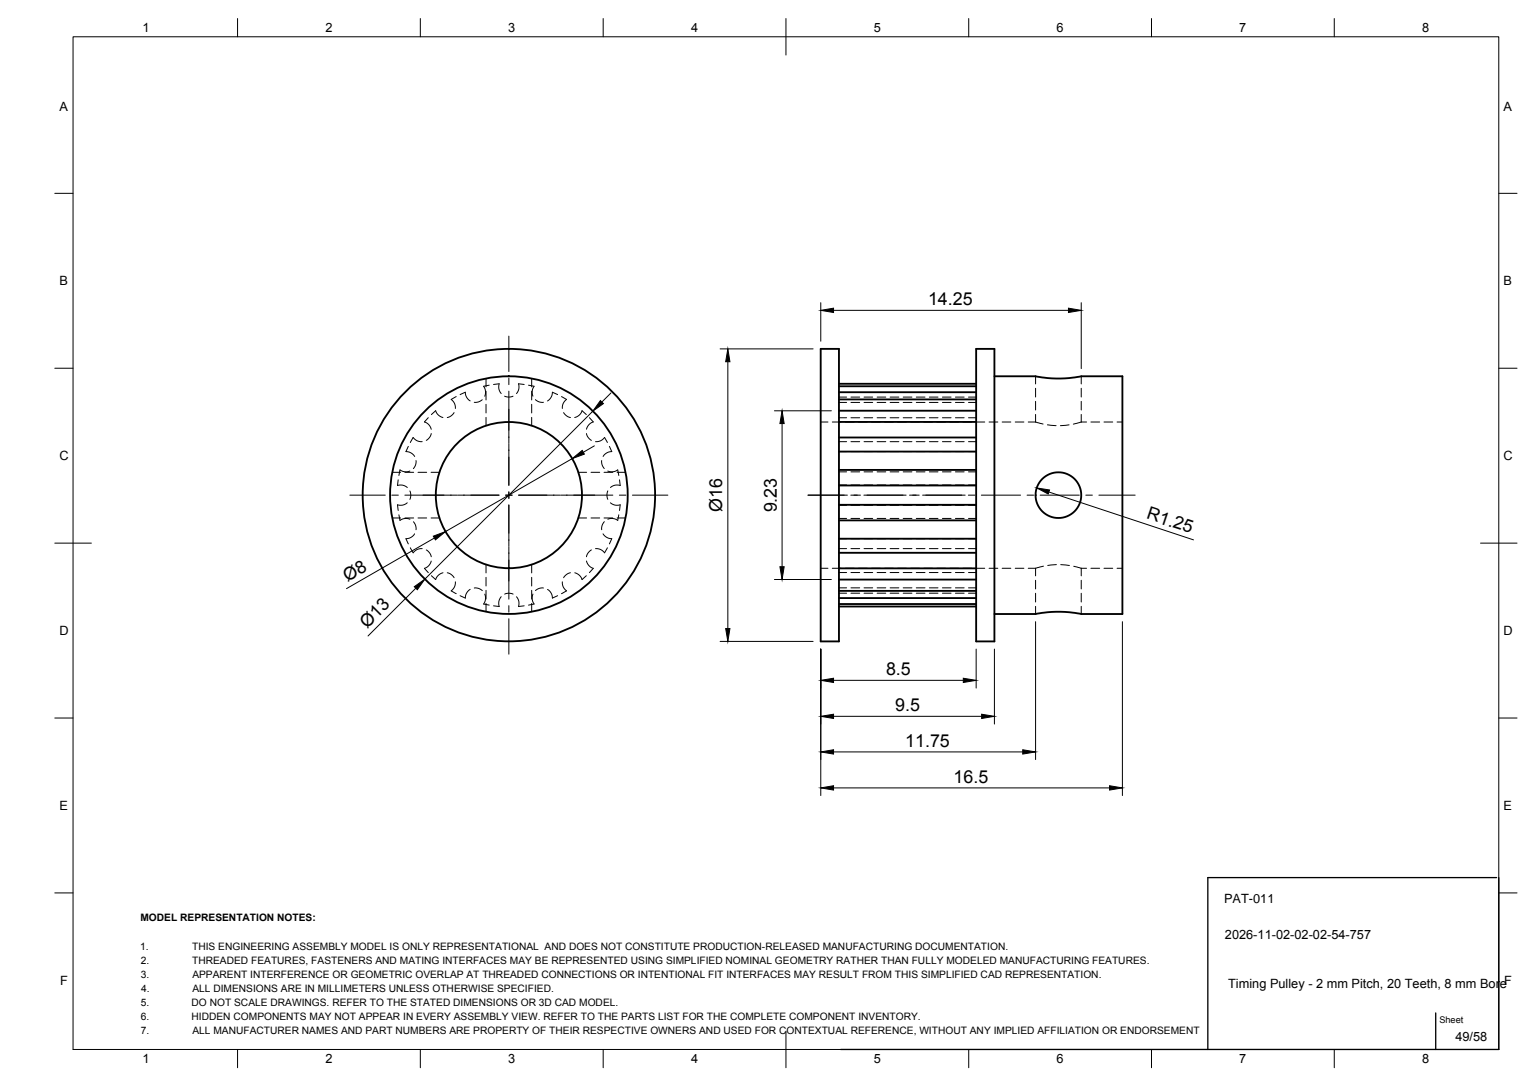
ISO-10303-21;
HEADER;
/* Generated by software containing ST-Developer
 * from STEP Tools, Inc. (www.steptools.com) 
 */

FILE_DESCRIPTION(
/* description */ ('Belt tension measurement rig'),
/* implementation_level */ '2;1');

FILE_NAME(
/* name */ 'Timing Pulley - 2 mm Pitch, 20 Teeth, 8 mm Bore.step',
/* time_stamp */ '2026-10-28T03:24:44-07:00',
/* author */ (''),
/* organization */ (''),
/* preprocessor_version */ 'ST-DEVELOPER v20.2',
/* originating_system */ 'Autodesk Translation Framework v15.17.0.0',
/* authorisation */ '');

FILE_SCHEMA (('AUTOMOTIVE_DESIGN { 1 0 10303 214 3 1 1 }'));
ENDSEC;

DATA;
#10=MECHANICAL_DESIGN_GEOMETRIC_PRESENTATION_REPRESENTATION('',(#750),#23587);
#531=B_SPLINE_CURVE_WITH_KNOTS('',3,(#21553,#21554,#21555,#21556,#21557,
#21558,#21559,#21560,#21561,#21562),.UNSPECIFIED.,.F.,.F.,(4,2,2,2,4),(0.566550474129931,
0.613761886174531,0.66097329821913,0.708186965196186,0.755400632173242),
 .UNSPECIFIED.);
#532=B_SPLINE_CURVE_WITH_KNOTS('',3,(#21564,#21565,#21566,#21567,#21568,
#21569,#21570,#21571,#21572,#21573,#21574,#21575,#21576,#21577,#21578,#21579,
#21580,#21581),.UNSPECIFIED.,.F.,.F.,(4,2,2,2,2,2,2,2,4),(0.18885015804331,
0.23606157008791,0.283272982132509,0.330486649109565,0.377700316086621,
0.424913983063677,0.472127650040732,0.519339062085332,0.566550474129931),
 .UNSPECIFIED.);
#533=B_SPLINE_CURVE_WITH_KNOTS('',3,(#21582,#21583,#21584,#21585,#21586,
#21587,#21588,#21589,#21590,#21591),.UNSPECIFIED.,.F.,.F.,(4,2,2,2,4),(0.755400632173242,
0.802614299150298,0.849827966127353,0.897039378171953,0.944250790216552),
 .UNSPECIFIED.);
#534=B_SPLINE_CURVE_WITH_KNOTS('',3,(#21595,#21596,#21597,#21598,#21599,
#21600,#21601,#21602,#21603,#21604),.UNSPECIFIED.,.F.,.F.,(4,2,2,2,4),(0.189723673274825,
0.237146208024627,0.28456874277443,0.33200804466204,0.37944734654965),
 .UNSPECIFIED.);
#535=B_SPLINE_CURVE_WITH_KNOTS('',3,(#21606,#21607,#21608,#21609,#21610,
#21611,#21612,#21613,#21614,#21615),.UNSPECIFIED.,.F.,.F.,(4,2,2,2,4),(0.,
0.0474393018876097,0.0948786037752193,0.142301138525022,0.189723673274825),
 .UNSPECIFIED.);
#536=B_SPLINE_CURVE_WITH_KNOTS('',3,(#21617,#21618,#21619,#21620,#21621,
#21622,#21623,#21624,#21625,#21626),.UNSPECIFIED.,.F.,.F.,(4,2,2,2,4),(0.569171019824474,
0.616593554574277,0.66401608932408,0.711455391211689,0.758894693099299),
 .UNSPECIFIED.);
#537=B_SPLINE_CURVE_WITH_KNOTS('',3,(#21627,#21628,#21629,#21630,#21631,
#21632,#21633,#21634,#21635,#21636),.UNSPECIFIED.,.F.,.F.,(4,2,2,2,4),(0.37944734654965,
0.426886648437259,0.474325950324869,0.521748485074671,0.569171019824474),
 .UNSPECIFIED.);
#538=B_SPLINE_CURVE_WITH_KNOTS('',3,(#21640,#21641,#21642,#21643,#21644,
#21645,#21646,#21647,#21648,#21649,#21650,#21651,#21652,#21653,#21654,#21655,
#21656,#21657),.UNSPECIFIED.,.F.,.F.,(4,2,2,2,2,2,2,2,4),(0.,0.0474393018876097,
0.0948786037752194,0.142301138525022,0.189723673274825,0.237146208024628,
0.28456874277443,0.33200804466204,0.37944734654965),.UNSPECIFIED.);
#539=B_SPLINE_CURVE_WITH_KNOTS('',3,(#21658,#21659,#21660,#21661,#21662,
#21663,#21664,#21665,#21666,#21667,#21668,#21669,#21670,#21671,#21672,#21673,
#21674,#21675),.UNSPECIFIED.,.F.,.F.,(4,2,2,2,2,2,2,2,4),(0.37944734654965,
0.426886648437259,0.474325950324869,0.521748485074672,0.569171019824474,
0.616593554574277,0.66401608932408,0.711455391211689,0.758894693099299),
 .UNSPECIFIED.);
#540=B_SPLINE_CURVE_WITH_KNOTS('',3,(#21679,#21680,#21681,#21682,#21683,
#21684,#21685,#21686,#21687,#21688),.UNSPECIFIED.,.F.,.F.,(4,2,2,2,4),(0.566550474129931,
0.613761886174531,0.66097329821913,0.708186965196186,0.755400632173242),
 .UNSPECIFIED.);
#541=B_SPLINE_CURVE_WITH_KNOTS('',3,(#21690,#21691,#21692,#21693,#21694,
#21695,#21696,#21697,#21698,#21699,#21700,#21701,#21702,#21703,#21704,#21705,
#21706,#21707),.UNSPECIFIED.,.F.,.F.,(4,2,2,2,2,2,2,2,4),(0.188850158043311,
0.23606157008791,0.283272982132509,0.330486649109565,0.377700316086621,
0.424913983063677,0.472127650040733,0.519339062085332,0.566550474129931),
 .UNSPECIFIED.);
#542=B_SPLINE_CURVE_WITH_KNOTS('',3,(#21708,#21709,#21710,#21711,#21712,
#21713,#21714,#21715,#21716,#21717),.UNSPECIFIED.,.F.,.F.,(4,2,2,2,4),(0.755400632173242,
0.802614299150298,0.849827966127354,0.897039378171953,0.944250790216552),
 .UNSPECIFIED.);
#543=B_SPLINE_CURVE_WITH_KNOTS('',3,(#21727,#21728,#21729,#21730,#21731,
#21732,#21733,#21734,#21735,#21736,#21737,#21738,#21739,#21740,#21741,#21742,
#21743,#21744),.UNSPECIFIED.,.F.,.F.,(4,2,2,2,2,2,2,2,4),(0.18885015804331,
0.23606157008791,0.283272982132509,0.330486649109565,0.377700316086621,
0.424913983063677,0.472127650040732,0.519339062085332,0.566550474129931),
 .UNSPECIFIED.);
#544=B_SPLINE_CURVE_WITH_KNOTS('',3,(#21746,#21747,#21748,#21749,#21750,
#21751,#21752,#21753,#21754,#21755),.UNSPECIFIED.,.F.,.F.,(4,2,2,2,4),(0.566550474129931,
0.613761886174531,0.66097329821913,0.708186965196186,0.755400632173242),
 .UNSPECIFIED.);
#545=B_SPLINE_CURVE_WITH_KNOTS('',3,(#21756,#21757,#21758,#21759,#21760,
#21761,#21762,#21763,#21764,#21765),.UNSPECIFIED.,.F.,.F.,(4,2,2,2,4),(0.755400632173242,
0.802614299150298,0.849827966127353,0.897039378171953,0.944250790216552),
 .UNSPECIFIED.);
#546=B_SPLINE_CURVE_WITH_KNOTS('',3,(#21768,#21769,#21770,#21771,#21772,
#21773,#21774,#21775,#21776,#21777,#21778,#21779,#21780,#21781,#21782,#21783,
#21784,#21785),.UNSPECIFIED.,.F.,.F.,(4,2,2,2,2,2,2,2,4),(0.188850158043311,
0.23606157008791,0.283272982132509,0.330486649109565,0.377700316086621,
0.424913983063677,0.472127650040733,0.519339062085332,0.566550474129932),
 .UNSPECIFIED.);
#547=B_SPLINE_CURVE_WITH_KNOTS('',3,(#21787,#21788,#21789,#21790,#21791,
#21792,#21793,#21794,#21795,#21796),.UNSPECIFIED.,.F.,.F.,(4,2,2,2,4),(0.566550474129932,
0.613761886174531,0.66097329821913,0.708186965196186,0.755400632173242),
 .UNSPECIFIED.);
#548=B_SPLINE_CURVE_WITH_KNOTS('',3,(#21797,#21798,#21799,#21800,#21801,
#21802,#21803,#21804,#21805,#21806),.UNSPECIFIED.,.F.,.F.,(4,2,2,2,4),(0.755400632173242,
0.802614299150298,0.849827966127354,0.897039378171953,0.944250790216552),
 .UNSPECIFIED.);
#549=B_SPLINE_CURVE_WITH_KNOTS('',3,(#21811,#21812,#21813,#21814,#21815,
#21816,#21817,#21818,#21819,#21820,#21821,#21822,#21823,#21824,#21825,#21826,
#21827,#21828),.UNSPECIFIED.,.F.,.F.,(4,2,2,2,2,2,2,2,4),(0.,0.0474393018876097,
0.0948786037752193,0.142301138525022,0.189723673274825,0.237146208024627,
0.28456874277443,0.33200804466204,0.37944734654965),.UNSPECIFIED.);
#550=B_SPLINE_CURVE_WITH_KNOTS('',3,(#21829,#21830,#21831,#21832,#21833,
#21834,#21835,#21836,#21837,#21838,#21839,#21840,#21841,#21842,#21843,#21844,
#21845,#21846),.UNSPECIFIED.,.F.,.F.,(4,2,2,2,2,2,2,2,4),(0.37944734654965,
0.426886648437259,0.474325950324869,0.521748485074672,0.569171019824474,
0.616593554574277,0.66401608932408,0.711455391211689,0.758894693099299),
 .UNSPECIFIED.);
#551=B_SPLINE_CURVE_WITH_KNOTS('',3,(#21850,#21851,#21852,#21853,#21854,
#21855,#21856,#21857,#21858,#21859,#21860,#21861,#21862,#21863,#21864,#21865,
#21866,#21867),.UNSPECIFIED.,.F.,.F.,(4,2,2,2,2,2,2,2,4),(0.,0.0474393018876097,
0.0948786037752194,0.142301138525022,0.189723673274825,0.237146208024627,
0.28456874277443,0.33200804466204,0.37944734654965),.UNSPECIFIED.);
#552=B_SPLINE_CURVE_WITH_KNOTS('',3,(#21868,#21869,#21870,#21871,#21872,
#21873,#21874,#21875,#21876,#21877,#21878,#21879,#21880,#21881,#21882,#21883,
#21884,#21885),.UNSPECIFIED.,.F.,.F.,(4,2,2,2,2,2,2,2,4),(0.37944734654965,
0.426886648437259,0.474325950324869,0.521748485074672,0.569171019824474,
0.616593554574277,0.66401608932408,0.711455391211689,0.758894693099299),
 .UNSPECIFIED.);
#625=SHAPE_REPRESENTATION_RELATIONSHIP('SRR','None',#23875,#680);
#680=ADVANCED_BREP_SHAPE_REPRESENTATION('',(#818),#23573);
#750=STYLED_ITEM('',(#24225),#818);
#818=MANIFOLD_SOLID_BREP('Body1',#12257);
#995=FACE_BOUND('',#2703,.T.);
#996=FACE_BOUND('',#2704,.T.);
#997=FACE_BOUND('',#2705,.T.);
#998=FACE_BOUND('',#2709,.T.);
#999=FACE_BOUND('',#2710,.T.);
#1000=FACE_BOUND('',#2711,.T.);
#1001=FACE_BOUND('',#2713,.T.);
#1002=FACE_BOUND('',#2715,.T.);
#1003=FACE_BOUND('',#2718,.T.);
#1004=FACE_BOUND('',#2720,.T.);
#1005=FACE_BOUND('',#2723,.T.);
#1294=PLANE('',#13882);
#1295=PLANE('',#13883);
#1296=PLANE('',#13927);
#1297=PLANE('',#13928);
#1298=PLANE('',#13972);
#1830=FACE_OUTER_BOUND('',#2700,.T.);
#1831=FACE_OUTER_BOUND('',#2701,.T.);
#1832=FACE_OUTER_BOUND('',#2702,.T.);
#1833=FACE_OUTER_BOUND('',#2706,.T.);
#1834=FACE_OUTER_BOUND('',#2707,.T.);
#1835=FACE_OUTER_BOUND('',#2708,.T.);
#1836=FACE_OUTER_BOUND('',#2712,.T.);
#1837=FACE_OUTER_BOUND('',#2714,.T.);
#1838=FACE_OUTER_BOUND('',#2716,.T.);
#1839=FACE_OUTER_BOUND('',#2717,.T.);
#1840=FACE_OUTER_BOUND('',#2719,.T.);
#1841=FACE_OUTER_BOUND('',#2721,.T.);
#1842=FACE_OUTER_BOUND('',#2722,.T.);
#1843=FACE_OUTER_BOUND('',#2724,.T.);
#1844=FACE_OUTER_BOUND('',#2725,.T.);
#1845=FACE_OUTER_BOUND('',#2726,.T.);
#1846=FACE_OUTER_BOUND('',#2727,.T.);
#1847=FACE_OUTER_BOUND('',#2728,.T.);
#1848=FACE_OUTER_BOUND('',#2729,.T.);
#1849=FACE_OUTER_BOUND('',#2730,.T.);
#1850=FACE_OUTER_BOUND('',#2731,.T.);
#1851=FACE_OUTER_BOUND('',#2732,.T.);
#1852=FACE_OUTER_BOUND('',#2733,.T.);
#1853=FACE_OUTER_BOUND('',#2734,.T.);
#1854=FACE_OUTER_BOUND('',#2735,.T.);
#1855=FACE_OUTER_BOUND('',#2736,.T.);
#1856=FACE_OUTER_BOUND('',#2737,.T.);
#1857=FACE_OUTER_BOUND('',#2738,.T.);
#1858=FACE_OUTER_BOUND('',#2739,.T.);
#1859=FACE_OUTER_BOUND('',#2740,.T.);
#1860=FACE_OUTER_BOUND('',#2741,.T.);
#1861=FACE_OUTER_BOUND('',#2742,.T.);
#1862=FACE_OUTER_BOUND('',#2743,.T.);
#1863=FACE_OUTER_BOUND('',#2744,.T.);
#1864=FACE_OUTER_BOUND('',#2745,.T.);
#1865=FACE_OUTER_BOUND('',#2746,.T.);
#1866=FACE_OUTER_BOUND('',#2747,.T.);
#1867=FACE_OUTER_BOUND('',#2748,.T.);
#1868=FACE_OUTER_BOUND('',#2749,.T.);
#1869=FACE_OUTER_BOUND('',#2750,.T.);
#1870=FACE_OUTER_BOUND('',#2751,.T.);
#1871=FACE_OUTER_BOUND('',#2752,.T.);
#1872=FACE_OUTER_BOUND('',#2753,.T.);
#1873=FACE_OUTER_BOUND('',#2754,.T.);
#1874=FACE_OUTER_BOUND('',#2755,.T.);
#1875=FACE_OUTER_BOUND('',#2756,.T.);
#1876=FACE_OUTER_BOUND('',#2757,.T.);
#1877=FACE_OUTER_BOUND('',#2758,.T.);
#1878=FACE_OUTER_BOUND('',#2759,.T.);
#1879=FACE_OUTER_BOUND('',#2760,.T.);
#1880=FACE_OUTER_BOUND('',#2761,.T.);
#1881=FACE_OUTER_BOUND('',#2762,.T.);
#1882=FACE_OUTER_BOUND('',#2763,.T.);
#2700=EDGE_LOOP('',(#10004,#10005,#10006,#10007,#10008,#10009,#10010,#10011,
#10012));
#2701=EDGE_LOOP('',(#10013,#10014,#10015,#10016,#10017,#10018,#10019));
#2702=EDGE_LOOP('',(#10020,#10021,#10022,#10023,#10024,#10025,#10026,#10027,
#10028));
#2703=EDGE_LOOP('',(#10029,#10030,#10031));
#2704=EDGE_LOOP('',(#10032,#10033,#10034));
#2705=EDGE_LOOP('',(#10035,#10036,#10037));
#2706=EDGE_LOOP('',(#10038,#10039,#10040,#10041,#10042,#10043,#10044));
#2707=EDGE_LOOP('',(#10045,#10046,#10047,#10048,#10049,#10050,#10051));
#2708=EDGE_LOOP('',(#10052,#10053,#10054,#10055,#10056,#10057,#10058,#10059,
#10060,#10061));
#2709=EDGE_LOOP('',(#10062,#10063));
#2710=EDGE_LOOP('',(#10064,#10065));
#2711=EDGE_LOOP('',(#10066,#10067));
#2712=EDGE_LOOP('',(#10068));
#2713=EDGE_LOOP('',(#10069));
#2714=EDGE_LOOP('',(#10070));
#2715=EDGE_LOOP('',(#10071,#10072,#10073,#10074,#10075,#10076,#10077,#10078,
#10079,#10080,#10081,#10082,#10083,#10084,#10085,#10086,#10087,#10088,#10089,
#10090,#10091,#10092,#10093,#10094,#10095,#10096,#10097,#10098,#10099,#10100,
#10101,#10102,#10103,#10104,#10105,#10106,#10107,#10108,#10109,#10110));
#2716=EDGE_LOOP('',(#10111,#10112,#10113,#10114));
#2717=EDGE_LOOP('',(#10115));
#2718=EDGE_LOOP('',(#10116));
#2719=EDGE_LOOP('',(#10117));
#2720=EDGE_LOOP('',(#10118,#10119,#10120,#10121,#10122,#10123,#10124,#10125,
#10126,#10127,#10128,#10129,#10130,#10131,#10132,#10133,#10134,#10135,#10136,
#10137,#10138,#10139,#10140,#10141,#10142,#10143,#10144,#10145,#10146,#10147,
#10148,#10149,#10150,#10151,#10152,#10153,#10154,#10155,#10156,#10157));
#2721=EDGE_LOOP('',(#10158,#10159,#10160,#10161));
#2722=EDGE_LOOP('',(#10162));
#2723=EDGE_LOOP('',(#10163));
#2724=EDGE_LOOP('',(#10164,#10165,#10166,#10167));
#2725=EDGE_LOOP('',(#10168,#10169,#10170,#10171));
#2726=EDGE_LOOP('',(#10172,#10173,#10174,#10175));
#2727=EDGE_LOOP('',(#10176,#10177,#10178,#10179));
#2728=EDGE_LOOP('',(#10180,#10181,#10182,#10183));
#2729=EDGE_LOOP('',(#10184,#10185,#10186,#10187));
#2730=EDGE_LOOP('',(#10188,#10189,#10190,#10191));
#2731=EDGE_LOOP('',(#10192,#10193,#10194,#10195));
#2732=EDGE_LOOP('',(#10196,#10197,#10198,#10199));
#2733=EDGE_LOOP('',(#10200,#10201,#10202,#10203));
#2734=EDGE_LOOP('',(#10204,#10205,#10206,#10207));
#2735=EDGE_LOOP('',(#10208,#10209,#10210,#10211));
#2736=EDGE_LOOP('',(#10212,#10213,#10214,#10215));
#2737=EDGE_LOOP('',(#10216,#10217,#10218,#10219));
#2738=EDGE_LOOP('',(#10220,#10221,#10222,#10223));
#2739=EDGE_LOOP('',(#10224,#10225,#10226,#10227));
#2740=EDGE_LOOP('',(#10228,#10229,#10230,#10231));
#2741=EDGE_LOOP('',(#10232,#10233,#10234,#10235));
#2742=EDGE_LOOP('',(#10236,#10237,#10238,#10239));
#2743=EDGE_LOOP('',(#10240,#10241,#10242,#10243));
#2744=EDGE_LOOP('',(#10244,#10245,#10246,#10247));
#2745=EDGE_LOOP('',(#10248,#10249,#10250,#10251));
#2746=EDGE_LOOP('',(#10252,#10253,#10254,#10255));
#2747=EDGE_LOOP('',(#10256,#10257,#10258,#10259));
#2748=EDGE_LOOP('',(#10260,#10261,#10262,#10263));
#2749=EDGE_LOOP('',(#10264,#10265,#10266,#10267));
#2750=EDGE_LOOP('',(#10268,#10269,#10270,#10271));
#2751=EDGE_LOOP('',(#10272,#10273,#10274,#10275));
#2752=EDGE_LOOP('',(#10276,#10277,#10278,#10279));
#2753=EDGE_LOOP('',(#10280,#10281,#10282,#10283));
#2754=EDGE_LOOP('',(#10284,#10285,#10286,#10287));
#2755=EDGE_LOOP('',(#10288,#10289,#10290,#10291));
#2756=EDGE_LOOP('',(#10292,#10293,#10294,#10295));
#2757=EDGE_LOOP('',(#10296,#10297,#10298,#10299));
#2758=EDGE_LOOP('',(#10300,#10301,#10302,#10303));
#2759=EDGE_LOOP('',(#10304,#10305,#10306,#10307));
#2760=EDGE_LOOP('',(#10308,#10309,#10310,#10311));
#2761=EDGE_LOOP('',(#10312,#10313,#10314,#10315));
#2762=EDGE_LOOP('',(#10316,#10317,#10318,#10319));
#2763=EDGE_LOOP('',(#10320,#10321,#10322,#10323));
#3507=LINE('',#21593,#4258);
#3508=LINE('',#21677,#4259);
#3509=LINE('',#21721,#4260);
#3510=LINE('',#21723,#4261);
#3511=LINE('',#21809,#4262);
#3512=LINE('',#21886,#4263);
#3513=LINE('',#21890,#4264);
#3514=LINE('',#21892,#4265);
#3515=LINE('',#21981,#4266);
#3516=LINE('',#22069,#4267);
#3517=LINE('',#22072,#4268);
#3518=LINE('',#22073,#4269);
#3519=LINE('',#22075,#4270);
#3520=LINE('',#22077,#4271);
#3521=LINE('',#22079,#4272);
#3522=LINE('',#22081,#4273);
#3523=LINE('',#22083,#4274);
#3524=LINE('',#22085,#4275);
#3525=LINE('',#22087,#4276);
#3526=LINE('',#22089,#4277);
#3527=LINE('',#22091,#4278);
#3528=LINE('',#22093,#4279);
#3529=LINE('',#22095,#4280);
#3530=LINE('',#22097,#4281);
#3531=LINE('',#22099,#4282);
#3532=LINE('',#22101,#4283);
#3533=LINE('',#22103,#4284);
#3534=LINE('',#22105,#4285);
#3535=LINE('',#22107,#4286);
#3536=LINE('',#22109,#4287);
#3537=LINE('',#22111,#4288);
#3538=LINE('',#22113,#4289);
#3539=LINE('',#22115,#4290);
#3540=LINE('',#22117,#4291);
#3541=LINE('',#22119,#4292);
#3542=LINE('',#22121,#4293);
#3543=LINE('',#22123,#4294);
#3544=LINE('',#22125,#4295);
#3545=LINE('',#22127,#4296);
#3546=LINE('',#22129,#4297);
#3547=LINE('',#22131,#4298);
#3548=LINE('',#22133,#4299);
#3549=LINE('',#22135,#4300);
#3550=LINE('',#22137,#4301);
#3551=LINE('',#22139,#4302);
#3552=LINE('',#22141,#4303);
#3553=LINE('',#22143,#4304);
#3554=LINE('',#22145,#4305);
#3555=LINE('',#22147,#4306);
#3556=LINE('',#22149,#4307);
#4258=VECTOR('',#17050,0.125);
#4259=VECTOR('',#17053,0.125);
#4260=VECTOR('',#17058,0.65);
#4261=VECTOR('',#17059,0.65);
#4262=VECTOR('',#17064,0.125);
#4263=VECTOR('',#17067,0.125);
#4264=VECTOR('',#17072,0.4);
#4265=VECTOR('',#17073,0.4);
#4266=VECTOR('',#17166,0.8);
#4267=VECTOR('',#17257,0.8);
#4268=VECTOR('',#17262,1.);
#4269=VECTOR('',#17263,1.);
#4270=VECTOR('',#17266,1.);
#4271=VECTOR('',#17269,1.);
#4272=VECTOR('',#17272,1.);
#4273=VECTOR('',#17275,1.);
#4274=VECTOR('',#17278,1.);
#4275=VECTOR('',#17281,1.);
#4276=VECTOR('',#17284,1.);
#4277=VECTOR('',#17287,1.);
#4278=VECTOR('',#17290,1.);
#4279=VECTOR('',#17293,1.);
#4280=VECTOR('',#17296,1.);
#4281=VECTOR('',#17299,1.);
#4282=VECTOR('',#17302,1.);
#4283=VECTOR('',#17305,1.);
#4284=VECTOR('',#17308,1.);
#4285=VECTOR('',#17311,1.);
#4286=VECTOR('',#17314,1.);
#4287=VECTOR('',#17317,1.);
#4288=VECTOR('',#17320,1.);
#4289=VECTOR('',#17323,1.);
#4290=VECTOR('',#17326,1.);
#4291=VECTOR('',#17329,1.);
#4292=VECTOR('',#17332,1.);
#4293=VECTOR('',#17335,1.);
#4294=VECTOR('',#17338,1.);
#4295=VECTOR('',#17341,1.);
#4296=VECTOR('',#17344,1.);
#4297=VECTOR('',#17347,1.);
#4298=VECTOR('',#17350,1.);
#4299=VECTOR('',#17353,1.);
#4300=VECTOR('',#17356,1.);
#4301=VECTOR('',#17359,1.);
#4302=VECTOR('',#17362,1.);
#4303=VECTOR('',#17365,1.);
#4304=VECTOR('',#17368,1.);
#4305=VECTOR('',#17371,1.);
#4306=VECTOR('',#17374,1.);
#4307=VECTOR('',#17377,1.);
#4924=CIRCLE('',#13875,0.65);
#4925=CIRCLE('',#13876,0.65);
#4926=CIRCLE('',#13880,0.4);
#4927=CIRCLE('',#13881,0.4);
#4928=CIRCLE('',#13884,0.8);
#4929=CIRCLE('',#13885,0.0555);
#4930=CIRCLE('',#13886,0.611219772367581);
#4931=CIRCLE('',#13887,0.0555);
#4932=CIRCLE('',#13888,0.611219772367581);
#4933=CIRCLE('',#13889,0.0555);
#4934=CIRCLE('',#13890,0.611219772367581);
#4935=CIRCLE('',#13891,0.0555);
#4936=CIRCLE('',#13892,0.611219772367581);
#4937=CIRCLE('',#13893,0.0555);
#4938=CIRCLE('',#13894,0.611219772367581);
#4939=CIRCLE('',#13895,0.0555);
#4940=CIRCLE('',#13896,0.611219772367581);
#4941=CIRCLE('',#13897,0.0555);
#4942=CIRCLE('',#13898,0.611219772367581);
#4943=CIRCLE('',#13899,0.0555);
#4944=CIRCLE('',#13900,0.611219772367581);
#4945=CIRCLE('',#13901,0.0555);
#4946=CIRCLE('',#13902,0.611219772367581);
#4947=CIRCLE('',#13903,0.0555);
#4948=CIRCLE('',#13904,0.611219772367581);
#4949=CIRCLE('',#13905,0.0555);
#4950=CIRCLE('',#13906,0.611219772367581);
#4951=CIRCLE('',#13907,0.0555);
#4952=CIRCLE('',#13908,0.611219772367581);
#4953=CIRCLE('',#13909,0.0555);
#4954=CIRCLE('',#13910,0.611219772367581);
#4955=CIRCLE('',#13911,0.0555);
#4956=CIRCLE('',#13912,0.611219772367581);
#4957=CIRCLE('',#13913,0.0555);
#4958=CIRCLE('',#13914,0.611219772367581);
#4959=CIRCLE('',#13915,0.0555);
#4960=CIRCLE('',#13916,0.611219772367581);
#4961=CIRCLE('',#13917,0.0555);
#4962=CIRCLE('',#13918,0.611219772367581);
#4963=CIRCLE('',#13919,0.0555);
#4964=CIRCLE('',#13920,0.611219772367581);
#4965=CIRCLE('',#13921,0.0555);
#4966=CIRCLE('',#13922,0.611219772367581);
#4967=CIRCLE('',#13923,0.0555);
#4968=CIRCLE('',#13924,0.611219772367581);
#4969=CIRCLE('',#13926,0.8);
#4970=CIRCLE('',#13929,0.8);
#4971=CIRCLE('',#13930,0.0555);
#4972=CIRCLE('',#13931,0.611219772367581);
#4973=CIRCLE('',#13932,0.0555);
#4974=CIRCLE('',#13933,0.611219772367581);
#4975=CIRCLE('',#13934,0.0555);
#4976=CIRCLE('',#13935,0.611219772367581);
#4977=CIRCLE('',#13936,0.0555);
#4978=CIRCLE('',#13937,0.611219772367581);
#4979=CIRCLE('',#13938,0.0555);
#4980=CIRCLE('',#13939,0.611219772367581);
#4981=CIRCLE('',#13940,0.0555);
#4982=CIRCLE('',#13941,0.611219772367581);
#4983=CIRCLE('',#13942,0.0555);
#4984=CIRCLE('',#13943,0.611219772367581);
#4985=CIRCLE('',#13944,0.0555);
#4986=CIRCLE('',#13945,0.611219772367581);
#4987=CIRCLE('',#13946,0.0555);
#4988=CIRCLE('',#13947,0.611219772367581);
#4989=CIRCLE('',#13948,0.0555);
#4990=CIRCLE('',#13949,0.611219772367581);
#4991=CIRCLE('',#13950,0.0555);
#4992=CIRCLE('',#13951,0.611219772367581);
#4993=CIRCLE('',#13952,0.0555);
#4994=CIRCLE('',#13953,0.611219772367581);
#4995=CIRCLE('',#13954,0.0555);
#4996=CIRCLE('',#13955,0.611219772367581);
#4997=CIRCLE('',#13956,0.0555);
#4998=CIRCLE('',#13957,0.611219772367581);
#4999=CIRCLE('',#13958,0.0555);
#5000=CIRCLE('',#13959,0.611219772367581);
#5001=CIRCLE('',#13960,0.0555);
#5002=CIRCLE('',#13961,0.611219772367581);
#5003=CIRCLE('',#13962,0.0555);
#5004=CIRCLE('',#13963,0.611219772367581);
#5005=CIRCLE('',#13964,0.0555);
#5006=CIRCLE('',#13965,0.611219772367581);
#5007=CIRCLE('',#13966,0.0555);
#5008=CIRCLE('',#13967,0.611219772367581);
#5009=CIRCLE('',#13968,0.0555);
#5010=CIRCLE('',#13969,0.611219772367581);
#5011=CIRCLE('',#13971,0.8);
#5939=VERTEX_POINT('',#21551);
#5940=VERTEX_POINT('',#21552);
#5941=VERTEX_POINT('',#21563);
#5942=VERTEX_POINT('',#21592);
#5943=VERTEX_POINT('',#21594);
#5944=VERTEX_POINT('',#21605);
#5945=VERTEX_POINT('',#21616);
#5946=VERTEX_POINT('',#21638);
#5947=VERTEX_POINT('',#21639);
#5948=VERTEX_POINT('',#21676);
#5949=VERTEX_POINT('',#21678);
#5950=VERTEX_POINT('',#21689);
#5951=VERTEX_POINT('',#21719);
#5952=VERTEX_POINT('',#21722);
#5953=VERTEX_POINT('',#21725);
#5954=VERTEX_POINT('',#21726);
#5955=VERTEX_POINT('',#21745);
#5956=VERTEX_POINT('',#21766);
#5957=VERTEX_POINT('',#21767);
#5958=VERTEX_POINT('',#21786);
#5959=VERTEX_POINT('',#21808);
#5960=VERTEX_POINT('',#21810);
#5961=VERTEX_POINT('',#21848);
#5962=VERTEX_POINT('',#21849);
#5963=VERTEX_POINT('',#21888);
#5964=VERTEX_POINT('',#21891);
#5965=VERTEX_POINT('',#21896);
#5966=VERTEX_POINT('',#21898);
#5967=VERTEX_POINT('',#21899);
#5968=VERTEX_POINT('',#21901);
#5969=VERTEX_POINT('',#21903);
#5970=VERTEX_POINT('',#21905);
#5971=VERTEX_POINT('',#21907);
#5972=VERTEX_POINT('',#21909);
#5973=VERTEX_POINT('',#21911);
#5974=VERTEX_POINT('',#21913);
#5975=VERTEX_POINT('',#21915);
#5976=VERTEX_POINT('',#21917);
#5977=VERTEX_POINT('',#21919);
#5978=VERTEX_POINT('',#21921);
#5979=VERTEX_POINT('',#21923);
#5980=VERTEX_POINT('',#21925);
#5981=VERTEX_POINT('',#21927);
#5982=VERTEX_POINT('',#21929);
#5983=VERTEX_POINT('',#21931);
#5984=VERTEX_POINT('',#21933);
#5985=VERTEX_POINT('',#21935);
#5986=VERTEX_POINT('',#21937);
#5987=VERTEX_POINT('',#21939);
#5988=VERTEX_POINT('',#21941);
#5989=VERTEX_POINT('',#21943);
#5990=VERTEX_POINT('',#21945);
#5991=VERTEX_POINT('',#21947);
#5992=VERTEX_POINT('',#21949);
#5993=VERTEX_POINT('',#21951);
#5994=VERTEX_POINT('',#21953);
#5995=VERTEX_POINT('',#21955);
#5996=VERTEX_POINT('',#21957);
#5997=VERTEX_POINT('',#21959);
#5998=VERTEX_POINT('',#21961);
#5999=VERTEX_POINT('',#21963);
#6000=VERTEX_POINT('',#21965);
#6001=VERTEX_POINT('',#21967);
#6002=VERTEX_POINT('',#21969);
#6003=VERTEX_POINT('',#21971);
#6004=VERTEX_POINT('',#21973);
#6005=VERTEX_POINT('',#21975);
#6006=VERTEX_POINT('',#21979);
#6007=VERTEX_POINT('',#21984);
#6008=VERTEX_POINT('',#21986);
#6009=VERTEX_POINT('',#21987);
#6010=VERTEX_POINT('',#21989);
#6011=VERTEX_POINT('',#21991);
#6012=VERTEX_POINT('',#21993);
#6013=VERTEX_POINT('',#21995);
#6014=VERTEX_POINT('',#21997);
#6015=VERTEX_POINT('',#21999);
#6016=VERTEX_POINT('',#22001);
#6017=VERTEX_POINT('',#22003);
#6018=VERTEX_POINT('',#22005);
#6019=VERTEX_POINT('',#22007);
#6020=VERTEX_POINT('',#22009);
#6021=VERTEX_POINT('',#22011);
#6022=VERTEX_POINT('',#22013);
#6023=VERTEX_POINT('',#22015);
#6024=VERTEX_POINT('',#22017);
#6025=VERTEX_POINT('',#22019);
#6026=VERTEX_POINT('',#22021);
#6027=VERTEX_POINT('',#22023);
#6028=VERTEX_POINT('',#22025);
#6029=VERTEX_POINT('',#22027);
#6030=VERTEX_POINT('',#22029);
#6031=VERTEX_POINT('',#22031);
#6032=VERTEX_POINT('',#22033);
#6033=VERTEX_POINT('',#22035);
#6034=VERTEX_POINT('',#22037);
#6035=VERTEX_POINT('',#22039);
#6036=VERTEX_POINT('',#22041);
#6037=VERTEX_POINT('',#22043);
#6038=VERTEX_POINT('',#22045);
#6039=VERTEX_POINT('',#22047);
#6040=VERTEX_POINT('',#22049);
#6041=VERTEX_POINT('',#22051);
#6042=VERTEX_POINT('',#22053);
#6043=VERTEX_POINT('',#22055);
#6044=VERTEX_POINT('',#22057);
#6045=VERTEX_POINT('',#22059);
#6046=VERTEX_POINT('',#22061);
#6047=VERTEX_POINT('',#22063);
#6048=VERTEX_POINT('',#22067);
#7361=EDGE_CURVE('',#5939,#5940,#531,.T.);
#7362=EDGE_CURVE('',#5941,#5939,#532,.T.);
#7363=EDGE_CURVE('',#5940,#5941,#533,.T.);
#7364=EDGE_CURVE('',#5940,#5942,#3507,.T.);
#7365=EDGE_CURVE('',#5943,#5942,#534,.T.);
#7366=EDGE_CURVE('',#5944,#5943,#535,.T.);
#7367=EDGE_CURVE('',#5945,#5944,#536,.T.);
#7368=EDGE_CURVE('',#5942,#5945,#537,.T.);
#7369=EDGE_CURVE('',#5946,#5947,#538,.T.);
#7370=EDGE_CURVE('',#5947,#5946,#539,.T.);
#7371=EDGE_CURVE('',#5947,#5948,#3508,.T.);
#7372=EDGE_CURVE('',#5949,#5948,#540,.T.);
#7373=EDGE_CURVE('',#5950,#5949,#541,.T.);
#7374=EDGE_CURVE('',#5948,#5950,#542,.T.);
#7375=EDGE_CURVE('',#5951,#5951,#4924,.T.);
#7376=EDGE_CURVE('',#5951,#5941,#3509,.T.);
#7377=EDGE_CURVE('',#5939,#5952,#3510,.T.);
#7378=EDGE_CURVE('',#5952,#5952,#4925,.T.);
#7379=EDGE_CURVE('',#5953,#5954,#543,.T.);
#7380=EDGE_CURVE('',#5954,#5955,#544,.T.);
#7381=EDGE_CURVE('',#5955,#5953,#545,.T.);
#7382=EDGE_CURVE('',#5956,#5957,#546,.T.);
#7383=EDGE_CURVE('',#5957,#5958,#547,.T.);
#7384=EDGE_CURVE('',#5958,#5956,#548,.T.);
#7385=EDGE_CURVE('',#5955,#5959,#3511,.T.);
#7386=EDGE_CURVE('',#5960,#5959,#549,.T.);
#7387=EDGE_CURVE('',#5959,#5960,#550,.T.);
#7388=EDGE_CURVE('',#5961,#5962,#551,.T.);
#7389=EDGE_CURVE('',#5962,#5961,#552,.T.);
#7390=EDGE_CURVE('',#5962,#5958,#3512,.T.);
#7391=EDGE_CURVE('',#5963,#5963,#4926,.T.);
#7392=EDGE_CURVE('',#5963,#5943,#3513,.T.);
#7393=EDGE_CURVE('',#5945,#5964,#3514,.T.);
#7394=EDGE_CURVE('',#5964,#5964,#4927,.T.);
#7395=EDGE_CURVE('',#5965,#5965,#4928,.T.);
#7396=EDGE_CURVE('',#5966,#5967,#4929,.T.);
#7397=EDGE_CURVE('',#5968,#5967,#4930,.T.);
#7398=EDGE_CURVE('',#5968,#5969,#4931,.T.);
#7399=EDGE_CURVE('',#5970,#5969,#4932,.T.);
#7400=EDGE_CURVE('',#5970,#5971,#4933,.T.);
#7401=EDGE_CURVE('',#5972,#5971,#4934,.T.);
#7402=EDGE_CURVE('',#5972,#5973,#4935,.T.);
#7403=EDGE_CURVE('',#5974,#5973,#4936,.T.);
#7404=EDGE_CURVE('',#5974,#5975,#4937,.T.);
#7405=EDGE_CURVE('',#5976,#5975,#4938,.T.);
#7406=EDGE_CURVE('',#5976,#5977,#4939,.T.);
#7407=EDGE_CURVE('',#5978,#5977,#4940,.T.);
#7408=EDGE_CURVE('',#5978,#5979,#4941,.T.);
#7409=EDGE_CURVE('',#5980,#5979,#4942,.T.);
#7410=EDGE_CURVE('',#5980,#5981,#4943,.T.);
#7411=EDGE_CURVE('',#5982,#5981,#4944,.T.);
#7412=EDGE_CURVE('',#5982,#5983,#4945,.T.);
#7413=EDGE_CURVE('',#5984,#5983,#4946,.T.);
#7414=EDGE_CURVE('',#5984,#5985,#4947,.T.);
#7415=EDGE_CURVE('',#5986,#5985,#4948,.T.);
#7416=EDGE_CURVE('',#5986,#5987,#4949,.T.);
#7417=EDGE_CURVE('',#5988,#5987,#4950,.T.);
#7418=EDGE_CURVE('',#5988,#5989,#4951,.T.);
#7419=EDGE_CURVE('',#5990,#5989,#4952,.T.);
#7420=EDGE_CURVE('',#5990,#5991,#4953,.T.);
#7421=EDGE_CURVE('',#5992,#5991,#4954,.T.);
#7422=EDGE_CURVE('',#5992,#5993,#4955,.T.);
#7423=EDGE_CURVE('',#5994,#5993,#4956,.T.);
#7424=EDGE_CURVE('',#5994,#5995,#4957,.T.);
#7425=EDGE_CURVE('',#5996,#5995,#4958,.T.);
#7426=EDGE_CURVE('',#5996,#5997,#4959,.T.);
#7427=EDGE_CURVE('',#5998,#5997,#4960,.T.);
#7428=EDGE_CURVE('',#5998,#5999,#4961,.T.);
#7429=EDGE_CURVE('',#6000,#5999,#4962,.T.);
#7430=EDGE_CURVE('',#6000,#6001,#4963,.T.);
#7431=EDGE_CURVE('',#6002,#6001,#4964,.T.);
#7432=EDGE_CURVE('',#6002,#6003,#4965,.T.);
#7433=EDGE_CURVE('',#6004,#6003,#4966,.T.);
#7434=EDGE_CURVE('',#6004,#6005,#4967,.T.);
#7435=EDGE_CURVE('',#5966,#6005,#4968,.T.);
#7436=EDGE_CURVE('',#6006,#6006,#4969,.T.);
#7437=EDGE_CURVE('',#6006,#5965,#3515,.T.);
#7438=EDGE_CURVE('',#6007,#6007,#4970,.T.);
#7439=EDGE_CURVE('',#6008,#6009,#4971,.T.);
#7440=EDGE_CURVE('',#6009,#6010,#4972,.T.);
#7441=EDGE_CURVE('',#6010,#6011,#4973,.T.);
#7442=EDGE_CURVE('',#6011,#6012,#4974,.T.);
#7443=EDGE_CURVE('',#6012,#6013,#4975,.T.);
#7444=EDGE_CURVE('',#6013,#6014,#4976,.T.);
#7445=EDGE_CURVE('',#6014,#6015,#4977,.T.);
#7446=EDGE_CURVE('',#6015,#6016,#4978,.T.);
#7447=EDGE_CURVE('',#6016,#6017,#4979,.T.);
#7448=EDGE_CURVE('',#6017,#6018,#4980,.T.);
#7449=EDGE_CURVE('',#6018,#6019,#4981,.T.);
#7450=EDGE_CURVE('',#6019,#6020,#4982,.T.);
#7451=EDGE_CURVE('',#6020,#6021,#4983,.T.);
#7452=EDGE_CURVE('',#6021,#6022,#4984,.T.);
#7453=EDGE_CURVE('',#6022,#6023,#4985,.T.);
#7454=EDGE_CURVE('',#6023,#6024,#4986,.T.);
#7455=EDGE_CURVE('',#6024,#6025,#4987,.T.);
#7456=EDGE_CURVE('',#6025,#6026,#4988,.T.);
#7457=EDGE_CURVE('',#6026,#6027,#4989,.T.);
#7458=EDGE_CURVE('',#6027,#6028,#4990,.T.);
#7459=EDGE_CURVE('',#6028,#6029,#4991,.T.);
#7460=EDGE_CURVE('',#6029,#6030,#4992,.T.);
#7461=EDGE_CURVE('',#6030,#6031,#4993,.T.);
#7462=EDGE_CURVE('',#6031,#6032,#4994,.T.);
#7463=EDGE_CURVE('',#6032,#6033,#4995,.T.);
#7464=EDGE_CURVE('',#6033,#6034,#4996,.T.);
#7465=EDGE_CURVE('',#6034,#6035,#4997,.T.);
#7466=EDGE_CURVE('',#6035,#6036,#4998,.T.);
#7467=EDGE_CURVE('',#6036,#6037,#4999,.T.);
#7468=EDGE_CURVE('',#6037,#6038,#5000,.T.);
#7469=EDGE_CURVE('',#6038,#6039,#5001,.T.);
#7470=EDGE_CURVE('',#6039,#6040,#5002,.T.);
#7471=EDGE_CURVE('',#6040,#6041,#5003,.T.);
#7472=EDGE_CURVE('',#6041,#6042,#5004,.T.);
#7473=EDGE_CURVE('',#6042,#6043,#5005,.T.);
#7474=EDGE_CURVE('',#6043,#6044,#5006,.T.);
#7475=EDGE_CURVE('',#6044,#6045,#5007,.T.);
#7476=EDGE_CURVE('',#6045,#6046,#5008,.T.);
#7477=EDGE_CURVE('',#6046,#6047,#5009,.T.);
#7478=EDGE_CURVE('',#6047,#6008,#5010,.T.);
#7479=EDGE_CURVE('',#6048,#6048,#5011,.T.);
#7480=EDGE_CURVE('',#6048,#6007,#3516,.T.);
#7481=EDGE_CURVE('',#6009,#5966,#3517,.T.);
#7482=EDGE_CURVE('',#5967,#6008,#3518,.T.);
#7483=EDGE_CURVE('',#6047,#5968,#3519,.T.);
#7484=EDGE_CURVE('',#5969,#6046,#3520,.T.);
#7485=EDGE_CURVE('',#6045,#5970,#3521,.T.);
#7486=EDGE_CURVE('',#5971,#6044,#3522,.T.);
#7487=EDGE_CURVE('',#6043,#5972,#3523,.T.);
#7488=EDGE_CURVE('',#5973,#6042,#3524,.T.);
#7489=EDGE_CURVE('',#6041,#5974,#3525,.T.);
#7490=EDGE_CURVE('',#5975,#6040,#3526,.T.);
#7491=EDGE_CURVE('',#6039,#5976,#3527,.T.);
#7492=EDGE_CURVE('',#5977,#6038,#3528,.T.);
#7493=EDGE_CURVE('',#6037,#5978,#3529,.T.);
#7494=EDGE_CURVE('',#5979,#6036,#3530,.T.);
#7495=EDGE_CURVE('',#6035,#5980,#3531,.T.);
#7496=EDGE_CURVE('',#5981,#6034,#3532,.T.);
#7497=EDGE_CURVE('',#6033,#5982,#3533,.T.);
#7498=EDGE_CURVE('',#5983,#6032,#3534,.T.);
#7499=EDGE_CURVE('',#6031,#5984,#3535,.T.);
#7500=EDGE_CURVE('',#5985,#6030,#3536,.T.);
#7501=EDGE_CURVE('',#6029,#5986,#3537,.T.);
#7502=EDGE_CURVE('',#5987,#6028,#3538,.T.);
#7503=EDGE_CURVE('',#6027,#5988,#3539,.T.);
#7504=EDGE_CURVE('',#5989,#6026,#3540,.T.);
#7505=EDGE_CURVE('',#6025,#5990,#3541,.T.);
#7506=EDGE_CURVE('',#5991,#6024,#3542,.T.);
#7507=EDGE_CURVE('',#6023,#5992,#3543,.T.);
#7508=EDGE_CURVE('',#5993,#6022,#3544,.T.);
#7509=EDGE_CURVE('',#6021,#5994,#3545,.T.);
#7510=EDGE_CURVE('',#5995,#6020,#3546,.T.);
#7511=EDGE_CURVE('',#6019,#5996,#3547,.T.);
#7512=EDGE_CURVE('',#5997,#6018,#3548,.T.);
#7513=EDGE_CURVE('',#6017,#5998,#3549,.T.);
#7514=EDGE_CURVE('',#5999,#6016,#3550,.T.);
#7515=EDGE_CURVE('',#6015,#6000,#3551,.T.);
#7516=EDGE_CURVE('',#6001,#6014,#3552,.T.);
#7517=EDGE_CURVE('',#6013,#6002,#3553,.T.);
#7518=EDGE_CURVE('',#6003,#6012,#3554,.T.);
#7519=EDGE_CURVE('',#6005,#6010,#3555,.T.);
#7520=EDGE_CURVE('',#6011,#6004,#3556,.T.);
#10004=ORIENTED_EDGE('',*,*,#7361,.F.);
#10005=ORIENTED_EDGE('',*,*,#7362,.F.);
#10006=ORIENTED_EDGE('',*,*,#7363,.F.);
#10007=ORIENTED_EDGE('',*,*,#7364,.T.);
#10008=ORIENTED_EDGE('',*,*,#7365,.F.);
#10009=ORIENTED_EDGE('',*,*,#7366,.F.);
#10010=ORIENTED_EDGE('',*,*,#7367,.F.);
#10011=ORIENTED_EDGE('',*,*,#7368,.F.);
#10012=ORIENTED_EDGE('',*,*,#7364,.F.);
#10013=ORIENTED_EDGE('',*,*,#7369,.F.);
#10014=ORIENTED_EDGE('',*,*,#7370,.F.);
#10015=ORIENTED_EDGE('',*,*,#7371,.T.);
#10016=ORIENTED_EDGE('',*,*,#7372,.F.);
#10017=ORIENTED_EDGE('',*,*,#7373,.F.);
#10018=ORIENTED_EDGE('',*,*,#7374,.F.);
#10019=ORIENTED_EDGE('',*,*,#7371,.F.);
#10020=ORIENTED_EDGE('',*,*,#7375,.F.);
#10021=ORIENTED_EDGE('',*,*,#7376,.T.);
#10022=ORIENTED_EDGE('',*,*,#7362,.T.);
#10023=ORIENTED_EDGE('',*,*,#7377,.T.);
#10024=ORIENTED_EDGE('',*,*,#7378,.F.);
#10025=ORIENTED_EDGE('',*,*,#7377,.F.);
#10026=ORIENTED_EDGE('',*,*,#7361,.T.);
#10027=ORIENTED_EDGE('',*,*,#7363,.T.);
#10028=ORIENTED_EDGE('',*,*,#7376,.F.);
#10029=ORIENTED_EDGE('',*,*,#7373,.T.);
#10030=ORIENTED_EDGE('',*,*,#7372,.T.);
#10031=ORIENTED_EDGE('',*,*,#7374,.T.);
#10032=ORIENTED_EDGE('',*,*,#7379,.T.);
#10033=ORIENTED_EDGE('',*,*,#7380,.T.);
#10034=ORIENTED_EDGE('',*,*,#7381,.T.);
#10035=ORIENTED_EDGE('',*,*,#7382,.T.);
#10036=ORIENTED_EDGE('',*,*,#7383,.T.);
#10037=ORIENTED_EDGE('',*,*,#7384,.T.);
#10038=ORIENTED_EDGE('',*,*,#7380,.F.);
#10039=ORIENTED_EDGE('',*,*,#7379,.F.);
#10040=ORIENTED_EDGE('',*,*,#7381,.F.);
#10041=ORIENTED_EDGE('',*,*,#7385,.T.);
#10042=ORIENTED_EDGE('',*,*,#7386,.F.);
#10043=ORIENTED_EDGE('',*,*,#7387,.F.);
#10044=ORIENTED_EDGE('',*,*,#7385,.F.);
#10045=ORIENTED_EDGE('',*,*,#7388,.F.);
#10046=ORIENTED_EDGE('',*,*,#7389,.F.);
#10047=ORIENTED_EDGE('',*,*,#7390,.T.);
#10048=ORIENTED_EDGE('',*,*,#7383,.F.);
#10049=ORIENTED_EDGE('',*,*,#7382,.F.);
#10050=ORIENTED_EDGE('',*,*,#7384,.F.);
#10051=ORIENTED_EDGE('',*,*,#7390,.F.);
#10052=ORIENTED_EDGE('',*,*,#7391,.F.);
#10053=ORIENTED_EDGE('',*,*,#7392,.T.);
#10054=ORIENTED_EDGE('',*,*,#7365,.T.);
#10055=ORIENTED_EDGE('',*,*,#7368,.T.);
#10056=ORIENTED_EDGE('',*,*,#7393,.T.);
#10057=ORIENTED_EDGE('',*,*,#7394,.F.);
#10058=ORIENTED_EDGE('',*,*,#7393,.F.);
#10059=ORIENTED_EDGE('',*,*,#7367,.T.);
#10060=ORIENTED_EDGE('',*,*,#7366,.T.);
#10061=ORIENTED_EDGE('',*,*,#7392,.F.);
#10062=ORIENTED_EDGE('',*,*,#7369,.T.);
#10063=ORIENTED_EDGE('',*,*,#7370,.T.);
#10064=ORIENTED_EDGE('',*,*,#7388,.T.);
#10065=ORIENTED_EDGE('',*,*,#7389,.T.);
#10066=ORIENTED_EDGE('',*,*,#7386,.T.);
#10067=ORIENTED_EDGE('',*,*,#7387,.T.);
#10068=ORIENTED_EDGE('',*,*,#7375,.T.);
#10069=ORIENTED_EDGE('',*,*,#7391,.T.);
#10070=ORIENTED_EDGE('',*,*,#7395,.T.);
#10071=ORIENTED_EDGE('',*,*,#7396,.T.);
#10072=ORIENTED_EDGE('',*,*,#7397,.F.);
#10073=ORIENTED_EDGE('',*,*,#7398,.T.);
#10074=ORIENTED_EDGE('',*,*,#7399,.F.);
#10075=ORIENTED_EDGE('',*,*,#7400,.T.);
#10076=ORIENTED_EDGE('',*,*,#7401,.F.);
#10077=ORIENTED_EDGE('',*,*,#7402,.T.);
#10078=ORIENTED_EDGE('',*,*,#7403,.F.);
#10079=ORIENTED_EDGE('',*,*,#7404,.T.);
#10080=ORIENTED_EDGE('',*,*,#7405,.F.);
#10081=ORIENTED_EDGE('',*,*,#7406,.T.);
#10082=ORIENTED_EDGE('',*,*,#7407,.F.);
#10083=ORIENTED_EDGE('',*,*,#7408,.T.);
#10084=ORIENTED_EDGE('',*,*,#7409,.F.);
#10085=ORIENTED_EDGE('',*,*,#7410,.T.);
#10086=ORIENTED_EDGE('',*,*,#7411,.F.);
#10087=ORIENTED_EDGE('',*,*,#7412,.T.);
#10088=ORIENTED_EDGE('',*,*,#7413,.F.);
#10089=ORIENTED_EDGE('',*,*,#7414,.T.);
#10090=ORIENTED_EDGE('',*,*,#7415,.F.);
#10091=ORIENTED_EDGE('',*,*,#7416,.T.);
#10092=ORIENTED_EDGE('',*,*,#7417,.F.);
#10093=ORIENTED_EDGE('',*,*,#7418,.T.);
#10094=ORIENTED_EDGE('',*,*,#7419,.F.);
#10095=ORIENTED_EDGE('',*,*,#7420,.T.);
#10096=ORIENTED_EDGE('',*,*,#7421,.F.);
#10097=ORIENTED_EDGE('',*,*,#7422,.T.);
#10098=ORIENTED_EDGE('',*,*,#7423,.F.);
#10099=ORIENTED_EDGE('',*,*,#7424,.T.);
#10100=ORIENTED_EDGE('',*,*,#7425,.F.);
#10101=ORIENTED_EDGE('',*,*,#7426,.T.);
#10102=ORIENTED_EDGE('',*,*,#7427,.F.);
#10103=ORIENTED_EDGE('',*,*,#7428,.T.);
#10104=ORIENTED_EDGE('',*,*,#7429,.F.);
#10105=ORIENTED_EDGE('',*,*,#7430,.T.);
#10106=ORIENTED_EDGE('',*,*,#7431,.F.);
#10107=ORIENTED_EDGE('',*,*,#7432,.T.);
#10108=ORIENTED_EDGE('',*,*,#7433,.F.);
#10109=ORIENTED_EDGE('',*,*,#7434,.T.);
#10110=ORIENTED_EDGE('',*,*,#7435,.F.);
#10111=ORIENTED_EDGE('',*,*,#7436,.F.);
#10112=ORIENTED_EDGE('',*,*,#7437,.T.);
#10113=ORIENTED_EDGE('',*,*,#7395,.F.);
#10114=ORIENTED_EDGE('',*,*,#7437,.F.);
#10115=ORIENTED_EDGE('',*,*,#7436,.T.);
#10116=ORIENTED_EDGE('',*,*,#7378,.T.);
#10117=ORIENTED_EDGE('',*,*,#7438,.F.);
#10118=ORIENTED_EDGE('',*,*,#7439,.T.);
#10119=ORIENTED_EDGE('',*,*,#7440,.T.);
#10120=ORIENTED_EDGE('',*,*,#7441,.T.);
#10121=ORIENTED_EDGE('',*,*,#7442,.T.);
#10122=ORIENTED_EDGE('',*,*,#7443,.T.);
#10123=ORIENTED_EDGE('',*,*,#7444,.T.);
#10124=ORIENTED_EDGE('',*,*,#7445,.T.);
#10125=ORIENTED_EDGE('',*,*,#7446,.T.);
#10126=ORIENTED_EDGE('',*,*,#7447,.T.);
#10127=ORIENTED_EDGE('',*,*,#7448,.T.);
#10128=ORIENTED_EDGE('',*,*,#7449,.T.);
#10129=ORIENTED_EDGE('',*,*,#7450,.T.);
#10130=ORIENTED_EDGE('',*,*,#7451,.T.);
#10131=ORIENTED_EDGE('',*,*,#7452,.T.);
#10132=ORIENTED_EDGE('',*,*,#7453,.T.);
#10133=ORIENTED_EDGE('',*,*,#7454,.T.);
#10134=ORIENTED_EDGE('',*,*,#7455,.T.);
#10135=ORIENTED_EDGE('',*,*,#7456,.T.);
#10136=ORIENTED_EDGE('',*,*,#7457,.T.);
#10137=ORIENTED_EDGE('',*,*,#7458,.T.);
#10138=ORIENTED_EDGE('',*,*,#7459,.T.);
#10139=ORIENTED_EDGE('',*,*,#7460,.T.);
#10140=ORIENTED_EDGE('',*,*,#7461,.T.);
#10141=ORIENTED_EDGE('',*,*,#7462,.T.);
#10142=ORIENTED_EDGE('',*,*,#7463,.T.);
#10143=ORIENTED_EDGE('',*,*,#7464,.T.);
#10144=ORIENTED_EDGE('',*,*,#7465,.T.);
#10145=ORIENTED_EDGE('',*,*,#7466,.T.);
#10146=ORIENTED_EDGE('',*,*,#7467,.T.);
#10147=ORIENTED_EDGE('',*,*,#7468,.T.);
#10148=ORIENTED_EDGE('',*,*,#7469,.T.);
#10149=ORIENTED_EDGE('',*,*,#7470,.T.);
#10150=ORIENTED_EDGE('',*,*,#7471,.T.);
#10151=ORIENTED_EDGE('',*,*,#7472,.T.);
#10152=ORIENTED_EDGE('',*,*,#7473,.T.);
#10153=ORIENTED_EDGE('',*,*,#7474,.T.);
#10154=ORIENTED_EDGE('',*,*,#7475,.T.);
#10155=ORIENTED_EDGE('',*,*,#7476,.T.);
#10156=ORIENTED_EDGE('',*,*,#7477,.T.);
#10157=ORIENTED_EDGE('',*,*,#7478,.T.);
#10158=ORIENTED_EDGE('',*,*,#7479,.F.);
#10159=ORIENTED_EDGE('',*,*,#7480,.T.);
#10160=ORIENTED_EDGE('',*,*,#7438,.T.);
#10161=ORIENTED_EDGE('',*,*,#7480,.F.);
#10162=ORIENTED_EDGE('',*,*,#7479,.T.);
#10163=ORIENTED_EDGE('',*,*,#7394,.T.);
#10164=ORIENTED_EDGE('',*,*,#7481,.F.);
#10165=ORIENTED_EDGE('',*,*,#7439,.F.);
#10166=ORIENTED_EDGE('',*,*,#7482,.F.);
#10167=ORIENTED_EDGE('',*,*,#7396,.F.);
#10168=ORIENTED_EDGE('',*,*,#7482,.T.);
#10169=ORIENTED_EDGE('',*,*,#7478,.F.);
#10170=ORIENTED_EDGE('',*,*,#7483,.T.);
#10171=ORIENTED_EDGE('',*,*,#7397,.T.);
#10172=ORIENTED_EDGE('',*,*,#7483,.F.);
#10173=ORIENTED_EDGE('',*,*,#7477,.F.);
#10174=ORIENTED_EDGE('',*,*,#7484,.F.);
#10175=ORIENTED_EDGE('',*,*,#7398,.F.);
#10176=ORIENTED_EDGE('',*,*,#7484,.T.);
#10177=ORIENTED_EDGE('',*,*,#7476,.F.);
#10178=ORIENTED_EDGE('',*,*,#7485,.T.);
#10179=ORIENTED_EDGE('',*,*,#7399,.T.);
#10180=ORIENTED_EDGE('',*,*,#7485,.F.);
#10181=ORIENTED_EDGE('',*,*,#7475,.F.);
#10182=ORIENTED_EDGE('',*,*,#7486,.F.);
#10183=ORIENTED_EDGE('',*,*,#7400,.F.);
#10184=ORIENTED_EDGE('',*,*,#7486,.T.);
#10185=ORIENTED_EDGE('',*,*,#7474,.F.);
#10186=ORIENTED_EDGE('',*,*,#7487,.T.);
#10187=ORIENTED_EDGE('',*,*,#7401,.T.);
#10188=ORIENTED_EDGE('',*,*,#7487,.F.);
#10189=ORIENTED_EDGE('',*,*,#7473,.F.);
#10190=ORIENTED_EDGE('',*,*,#7488,.F.);
#10191=ORIENTED_EDGE('',*,*,#7402,.F.);
#10192=ORIENTED_EDGE('',*,*,#7488,.T.);
#10193=ORIENTED_EDGE('',*,*,#7472,.F.);
#10194=ORIENTED_EDGE('',*,*,#7489,.T.);
#10195=ORIENTED_EDGE('',*,*,#7403,.T.);
#10196=ORIENTED_EDGE('',*,*,#7489,.F.);
#10197=ORIENTED_EDGE('',*,*,#7471,.F.);
#10198=ORIENTED_EDGE('',*,*,#7490,.F.);
#10199=ORIENTED_EDGE('',*,*,#7404,.F.);
#10200=ORIENTED_EDGE('',*,*,#7490,.T.);
#10201=ORIENTED_EDGE('',*,*,#7470,.F.);
#10202=ORIENTED_EDGE('',*,*,#7491,.T.);
#10203=ORIENTED_EDGE('',*,*,#7405,.T.);
#10204=ORIENTED_EDGE('',*,*,#7491,.F.);
#10205=ORIENTED_EDGE('',*,*,#7469,.F.);
#10206=ORIENTED_EDGE('',*,*,#7492,.F.);
#10207=ORIENTED_EDGE('',*,*,#7406,.F.);
#10208=ORIENTED_EDGE('',*,*,#7492,.T.);
#10209=ORIENTED_EDGE('',*,*,#7468,.F.);
#10210=ORIENTED_EDGE('',*,*,#7493,.T.);
#10211=ORIENTED_EDGE('',*,*,#7407,.T.);
#10212=ORIENTED_EDGE('',*,*,#7493,.F.);
#10213=ORIENTED_EDGE('',*,*,#7467,.F.);
#10214=ORIENTED_EDGE('',*,*,#7494,.F.);
#10215=ORIENTED_EDGE('',*,*,#7408,.F.);
#10216=ORIENTED_EDGE('',*,*,#7494,.T.);
#10217=ORIENTED_EDGE('',*,*,#7466,.F.);
#10218=ORIENTED_EDGE('',*,*,#7495,.T.);
#10219=ORIENTED_EDGE('',*,*,#7409,.T.);
#10220=ORIENTED_EDGE('',*,*,#7495,.F.);
#10221=ORIENTED_EDGE('',*,*,#7465,.F.);
#10222=ORIENTED_EDGE('',*,*,#7496,.F.);
#10223=ORIENTED_EDGE('',*,*,#7410,.F.);
#10224=ORIENTED_EDGE('',*,*,#7496,.T.);
#10225=ORIENTED_EDGE('',*,*,#7464,.F.);
#10226=ORIENTED_EDGE('',*,*,#7497,.T.);
#10227=ORIENTED_EDGE('',*,*,#7411,.T.);
#10228=ORIENTED_EDGE('',*,*,#7497,.F.);
#10229=ORIENTED_EDGE('',*,*,#7463,.F.);
#10230=ORIENTED_EDGE('',*,*,#7498,.F.);
#10231=ORIENTED_EDGE('',*,*,#7412,.F.);
#10232=ORIENTED_EDGE('',*,*,#7498,.T.);
#10233=ORIENTED_EDGE('',*,*,#7462,.F.);
#10234=ORIENTED_EDGE('',*,*,#7499,.T.);
#10235=ORIENTED_EDGE('',*,*,#7413,.T.);
#10236=ORIENTED_EDGE('',*,*,#7499,.F.);
#10237=ORIENTED_EDGE('',*,*,#7461,.F.);
#10238=ORIENTED_EDGE('',*,*,#7500,.F.);
#10239=ORIENTED_EDGE('',*,*,#7414,.F.);
#10240=ORIENTED_EDGE('',*,*,#7500,.T.);
#10241=ORIENTED_EDGE('',*,*,#7460,.F.);
#10242=ORIENTED_EDGE('',*,*,#7501,.T.);
#10243=ORIENTED_EDGE('',*,*,#7415,.T.);
#10244=ORIENTED_EDGE('',*,*,#7501,.F.);
#10245=ORIENTED_EDGE('',*,*,#7459,.F.);
#10246=ORIENTED_EDGE('',*,*,#7502,.F.);
#10247=ORIENTED_EDGE('',*,*,#7416,.F.);
#10248=ORIENTED_EDGE('',*,*,#7502,.T.);
#10249=ORIENTED_EDGE('',*,*,#7458,.F.);
#10250=ORIENTED_EDGE('',*,*,#7503,.T.);
#10251=ORIENTED_EDGE('',*,*,#7417,.T.);
#10252=ORIENTED_EDGE('',*,*,#7503,.F.);
#10253=ORIENTED_EDGE('',*,*,#7457,.F.);
#10254=ORIENTED_EDGE('',*,*,#7504,.F.);
#10255=ORIENTED_EDGE('',*,*,#7418,.F.);
#10256=ORIENTED_EDGE('',*,*,#7504,.T.);
#10257=ORIENTED_EDGE('',*,*,#7456,.F.);
#10258=ORIENTED_EDGE('',*,*,#7505,.T.);
#10259=ORIENTED_EDGE('',*,*,#7419,.T.);
#10260=ORIENTED_EDGE('',*,*,#7505,.F.);
#10261=ORIENTED_EDGE('',*,*,#7455,.F.);
#10262=ORIENTED_EDGE('',*,*,#7506,.F.);
#10263=ORIENTED_EDGE('',*,*,#7420,.F.);
#10264=ORIENTED_EDGE('',*,*,#7506,.T.);
#10265=ORIENTED_EDGE('',*,*,#7454,.F.);
#10266=ORIENTED_EDGE('',*,*,#7507,.T.);
#10267=ORIENTED_EDGE('',*,*,#7421,.T.);
#10268=ORIENTED_EDGE('',*,*,#7507,.F.);
#10269=ORIENTED_EDGE('',*,*,#7453,.F.);
#10270=ORIENTED_EDGE('',*,*,#7508,.F.);
#10271=ORIENTED_EDGE('',*,*,#7422,.F.);
#10272=ORIENTED_EDGE('',*,*,#7508,.T.);
#10273=ORIENTED_EDGE('',*,*,#7452,.F.);
#10274=ORIENTED_EDGE('',*,*,#7509,.T.);
#10275=ORIENTED_EDGE('',*,*,#7423,.T.);
#10276=ORIENTED_EDGE('',*,*,#7509,.F.);
#10277=ORIENTED_EDGE('',*,*,#7451,.F.);
#10278=ORIENTED_EDGE('',*,*,#7510,.F.);
#10279=ORIENTED_EDGE('',*,*,#7424,.F.);
#10280=ORIENTED_EDGE('',*,*,#7510,.T.);
#10281=ORIENTED_EDGE('',*,*,#7450,.F.);
#10282=ORIENTED_EDGE('',*,*,#7511,.T.);
#10283=ORIENTED_EDGE('',*,*,#7425,.T.);
#10284=ORIENTED_EDGE('',*,*,#7511,.F.);
#10285=ORIENTED_EDGE('',*,*,#7449,.F.);
#10286=ORIENTED_EDGE('',*,*,#7512,.F.);
#10287=ORIENTED_EDGE('',*,*,#7426,.F.);
#10288=ORIENTED_EDGE('',*,*,#7512,.T.);
#10289=ORIENTED_EDGE('',*,*,#7448,.F.);
#10290=ORIENTED_EDGE('',*,*,#7513,.T.);
#10291=ORIENTED_EDGE('',*,*,#7427,.T.);
#10292=ORIENTED_EDGE('',*,*,#7513,.F.);
#10293=ORIENTED_EDGE('',*,*,#7447,.F.);
#10294=ORIENTED_EDGE('',*,*,#7514,.F.);
#10295=ORIENTED_EDGE('',*,*,#7428,.F.);
#10296=ORIENTED_EDGE('',*,*,#7514,.T.);
#10297=ORIENTED_EDGE('',*,*,#7446,.F.);
#10298=ORIENTED_EDGE('',*,*,#7515,.T.);
#10299=ORIENTED_EDGE('',*,*,#7429,.T.);
#10300=ORIENTED_EDGE('',*,*,#7515,.F.);
#10301=ORIENTED_EDGE('',*,*,#7445,.F.);
#10302=ORIENTED_EDGE('',*,*,#7516,.F.);
#10303=ORIENTED_EDGE('',*,*,#7430,.F.);
#10304=ORIENTED_EDGE('',*,*,#7516,.T.);
#10305=ORIENTED_EDGE('',*,*,#7444,.F.);
#10306=ORIENTED_EDGE('',*,*,#7517,.T.);
#10307=ORIENTED_EDGE('',*,*,#7431,.T.);
#10308=ORIENTED_EDGE('',*,*,#7518,.F.);
#10309=ORIENTED_EDGE('',*,*,#7432,.F.);
#10310=ORIENTED_EDGE('',*,*,#7517,.F.);
#10311=ORIENTED_EDGE('',*,*,#7443,.F.);
#10312=ORIENTED_EDGE('',*,*,#7481,.T.);
#10313=ORIENTED_EDGE('',*,*,#7435,.T.);
#10314=ORIENTED_EDGE('',*,*,#7519,.T.);
#10315=ORIENTED_EDGE('',*,*,#7440,.F.);
#10316=ORIENTED_EDGE('',*,*,#7520,.F.);
#10317=ORIENTED_EDGE('',*,*,#7441,.F.);
#10318=ORIENTED_EDGE('',*,*,#7519,.F.);
#10319=ORIENTED_EDGE('',*,*,#7434,.F.);
#10320=ORIENTED_EDGE('',*,*,#7518,.T.);
#10321=ORIENTED_EDGE('',*,*,#7442,.F.);
#10322=ORIENTED_EDGE('',*,*,#7520,.T.);
#10323=ORIENTED_EDGE('',*,*,#7433,.T.);
#11331=CYLINDRICAL_SURFACE('',#13872,0.125);
#11332=CYLINDRICAL_SURFACE('',#13873,0.125);
#11333=CYLINDRICAL_SURFACE('',#13874,0.65);
#11334=CYLINDRICAL_SURFACE('',#13877,0.125);
#11335=CYLINDRICAL_SURFACE('',#13878,0.125);
#11336=CYLINDRICAL_SURFACE('',#13879,0.4);
#11337=CYLINDRICAL_SURFACE('',#13925,0.8);
#11338=CYLINDRICAL_SURFACE('',#13970,0.8);
#11339=CYLINDRICAL_SURFACE('',#13973,0.0555);
#11340=CYLINDRICAL_SURFACE('',#13974,0.611219772367581);
#11341=CYLINDRICAL_SURFACE('',#13975,0.0555);
#11342=CYLINDRICAL_SURFACE('',#13976,0.611219772367581);
#11343=CYLINDRICAL_SURFACE('',#13977,0.0555);
#11344=CYLINDRICAL_SURFACE('',#13978,0.611219772367581);
#11345=CYLINDRICAL_SURFACE('',#13979,0.0555);
#11346=CYLINDRICAL_SURFACE('',#13980,0.611219772367581);
#11347=CYLINDRICAL_SURFACE('',#13981,0.0555);
#11348=CYLINDRICAL_SURFACE('',#13982,0.611219772367581);
#11349=CYLINDRICAL_SURFACE('',#13983,0.0555);
#11350=CYLINDRICAL_SURFACE('',#13984,0.611219772367581);
#11351=CYLINDRICAL_SURFACE('',#13985,0.0555);
#11352=CYLINDRICAL_SURFACE('',#13986,0.611219772367581);
#11353=CYLINDRICAL_SURFACE('',#13987,0.0555);
#11354=CYLINDRICAL_SURFACE('',#13988,0.611219772367581);
#11355=CYLINDRICAL_SURFACE('',#13989,0.0555);
#11356=CYLINDRICAL_SURFACE('',#13990,0.611219772367581);
#11357=CYLINDRICAL_SURFACE('',#13991,0.0555);
#11358=CYLINDRICAL_SURFACE('',#13992,0.611219772367581);
#11359=CYLINDRICAL_SURFACE('',#13993,0.0555);
#11360=CYLINDRICAL_SURFACE('',#13994,0.611219772367581);
#11361=CYLINDRICAL_SURFACE('',#13995,0.0555);
#11362=CYLINDRICAL_SURFACE('',#13996,0.611219772367581);
#11363=CYLINDRICAL_SURFACE('',#13997,0.0555);
#11364=CYLINDRICAL_SURFACE('',#13998,0.611219772367581);
#11365=CYLINDRICAL_SURFACE('',#13999,0.0555);
#11366=CYLINDRICAL_SURFACE('',#14000,0.611219772367581);
#11367=CYLINDRICAL_SURFACE('',#14001,0.0555);
#11368=CYLINDRICAL_SURFACE('',#14002,0.611219772367581);
#11369=CYLINDRICAL_SURFACE('',#14003,0.0555);
#11370=CYLINDRICAL_SURFACE('',#14004,0.611219772367581);
#11371=CYLINDRICAL_SURFACE('',#14005,0.0555);
#11372=CYLINDRICAL_SURFACE('',#14006,0.611219772367581);
#11373=CYLINDRICAL_SURFACE('',#14007,0.0555);
#11374=CYLINDRICAL_SURFACE('',#14008,0.611219772367581);
#11375=CYLINDRICAL_SURFACE('',#14009,0.0555);
#11376=CYLINDRICAL_SURFACE('',#14010,0.611219772367581);
#11377=CYLINDRICAL_SURFACE('',#14011,0.0555);
#11378=CYLINDRICAL_SURFACE('',#14012,0.611219772367581);
#11971=ADVANCED_FACE('',(#1830),#11331,.F.);
#11972=ADVANCED_FACE('',(#1831),#11332,.F.);
#11973=ADVANCED_FACE('',(#1832,#995,#996,#997),#11333,.T.);
#11974=ADVANCED_FACE('',(#1833),#11334,.F.);
#11975=ADVANCED_FACE('',(#1834),#11335,.F.);
#11976=ADVANCED_FACE('',(#1835,#998,#999,#1000),#11336,.F.);
#11977=ADVANCED_FACE('',(#1836,#1001),#1294,.F.);
#11978=ADVANCED_FACE('',(#1837,#1002),#1295,.T.);
#11979=ADVANCED_FACE('',(#1838),#11337,.T.);
#11980=ADVANCED_FACE('',(#1839,#1003),#1296,.F.);
#11981=ADVANCED_FACE('',(#1840,#1004),#1297,.F.);
#11982=ADVANCED_FACE('',(#1841),#11338,.T.);
#11983=ADVANCED_FACE('',(#1842,#1005),#1298,.T.);
#11984=ADVANCED_FACE('',(#1843),#11339,.F.);
#11985=ADVANCED_FACE('',(#1844),#11340,.T.);
#11986=ADVANCED_FACE('',(#1845),#11341,.F.);
#11987=ADVANCED_FACE('',(#1846),#11342,.T.);
#11988=ADVANCED_FACE('',(#1847),#11343,.F.);
#11989=ADVANCED_FACE('',(#1848),#11344,.T.);
#11990=ADVANCED_FACE('',(#1849),#11345,.F.);
#11991=ADVANCED_FACE('',(#1850),#11346,.T.);
#11992=ADVANCED_FACE('',(#1851),#11347,.F.);
#11993=ADVANCED_FACE('',(#1852),#11348,.T.);
#11994=ADVANCED_FACE('',(#1853),#11349,.F.);
#11995=ADVANCED_FACE('',(#1854),#11350,.T.);
#11996=ADVANCED_FACE('',(#1855),#11351,.F.);
#11997=ADVANCED_FACE('',(#1856),#11352,.T.);
#11998=ADVANCED_FACE('',(#1857),#11353,.F.);
#11999=ADVANCED_FACE('',(#1858),#11354,.T.);
#12000=ADVANCED_FACE('',(#1859),#11355,.F.);
#12001=ADVANCED_FACE('',(#1860),#11356,.T.);
#12002=ADVANCED_FACE('',(#1861),#11357,.F.);
#12003=ADVANCED_FACE('',(#1862),#11358,.T.);
#12004=ADVANCED_FACE('',(#1863),#11359,.F.);
#12005=ADVANCED_FACE('',(#1864),#11360,.T.);
#12006=ADVANCED_FACE('',(#1865),#11361,.F.);
#12007=ADVANCED_FACE('',(#1866),#11362,.T.);
#12008=ADVANCED_FACE('',(#1867),#11363,.F.);
#12009=ADVANCED_FACE('',(#1868),#11364,.T.);
#12010=ADVANCED_FACE('',(#1869),#11365,.F.);
#12011=ADVANCED_FACE('',(#1870),#11366,.T.);
#12012=ADVANCED_FACE('',(#1871),#11367,.F.);
#12013=ADVANCED_FACE('',(#1872),#11368,.T.);
#12014=ADVANCED_FACE('',(#1873),#11369,.F.);
#12015=ADVANCED_FACE('',(#1874),#11370,.T.);
#12016=ADVANCED_FACE('',(#1875),#11371,.F.);
#12017=ADVANCED_FACE('',(#1876),#11372,.T.);
#12018=ADVANCED_FACE('',(#1877),#11373,.F.);
#12019=ADVANCED_FACE('',(#1878),#11374,.T.);
#12020=ADVANCED_FACE('',(#1879),#11375,.F.);
#12021=ADVANCED_FACE('',(#1880),#11376,.T.);
#12022=ADVANCED_FACE('',(#1881),#11377,.F.);
#12023=ADVANCED_FACE('',(#1882),#11378,.T.);
#12257=CLOSED_SHELL('',(#11971,#11972,#11973,#11974,#11975,#11976,#11977,
#11978,#11979,#11980,#11981,#11982,#11983,#11984,#11985,#11986,#11987,#11988,
#11989,#11990,#11991,#11992,#11993,#11994,#11995,#11996,#11997,#11998,#11999,
#12000,#12001,#12002,#12003,#12004,#12005,#12006,#12007,#12008,#12009,#12010,
#12011,#12012,#12013,#12014,#12015,#12016,#12017,#12018,#12019,#12020,#12021,
#12022,#12023));
#13871=AXIS2_PLACEMENT_3D('',#21549,#17046,#17047);
#13872=AXIS2_PLACEMENT_3D('',#21550,#17048,#17049);
#13873=AXIS2_PLACEMENT_3D('',#21637,#17051,#17052);
#13874=AXIS2_PLACEMENT_3D('',#21718,#17054,#17055);
#13875=AXIS2_PLACEMENT_3D('',#21720,#17056,#17057);
#13876=AXIS2_PLACEMENT_3D('',#21724,#17060,#17061);
#13877=AXIS2_PLACEMENT_3D('',#21807,#17062,#17063);
#13878=AXIS2_PLACEMENT_3D('',#21847,#17065,#17066);
#13879=AXIS2_PLACEMENT_3D('',#21887,#17068,#17069);
#13880=AXIS2_PLACEMENT_3D('',#21889,#17070,#17071);
#13881=AXIS2_PLACEMENT_3D('',#21893,#17074,#17075);
#13882=AXIS2_PLACEMENT_3D('',#21894,#17076,#17077);
#13883=AXIS2_PLACEMENT_3D('',#21895,#17078,#17079);
#13884=AXIS2_PLACEMENT_3D('',#21897,#17080,#17081);
#13885=AXIS2_PLACEMENT_3D('',#21900,#17082,#17083);
#13886=AXIS2_PLACEMENT_3D('',#21902,#17084,#17085);
#13887=AXIS2_PLACEMENT_3D('',#21904,#17086,#17087);
#13888=AXIS2_PLACEMENT_3D('',#21906,#17088,#17089);
#13889=AXIS2_PLACEMENT_3D('',#21908,#17090,#17091);
#13890=AXIS2_PLACEMENT_3D('',#21910,#17092,#17093);
#13891=AXIS2_PLACEMENT_3D('',#21912,#17094,#17095);
#13892=AXIS2_PLACEMENT_3D('',#21914,#17096,#17097);
#13893=AXIS2_PLACEMENT_3D('',#21916,#17098,#17099);
#13894=AXIS2_PLACEMENT_3D('',#21918,#17100,#17101);
#13895=AXIS2_PLACEMENT_3D('',#21920,#17102,#17103);
#13896=AXIS2_PLACEMENT_3D('',#21922,#17104,#17105);
#13897=AXIS2_PLACEMENT_3D('',#21924,#17106,#17107);
#13898=AXIS2_PLACEMENT_3D('',#21926,#17108,#17109);
#13899=AXIS2_PLACEMENT_3D('',#21928,#17110,#17111);
#13900=AXIS2_PLACEMENT_3D('',#21930,#17112,#17113);
#13901=AXIS2_PLACEMENT_3D('',#21932,#17114,#17115);
#13902=AXIS2_PLACEMENT_3D('',#21934,#17116,#17117);
#13903=AXIS2_PLACEMENT_3D('',#21936,#17118,#17119);
#13904=AXIS2_PLACEMENT_3D('',#21938,#17120,#17121);
#13905=AXIS2_PLACEMENT_3D('',#21940,#17122,#17123);
#13906=AXIS2_PLACEMENT_3D('',#21942,#17124,#17125);
#13907=AXIS2_PLACEMENT_3D('',#21944,#17126,#17127);
#13908=AXIS2_PLACEMENT_3D('',#21946,#17128,#17129);
#13909=AXIS2_PLACEMENT_3D('',#21948,#17130,#17131);
#13910=AXIS2_PLACEMENT_3D('',#21950,#17132,#17133);
#13911=AXIS2_PLACEMENT_3D('',#21952,#17134,#17135);
#13912=AXIS2_PLACEMENT_3D('',#21954,#17136,#17137);
#13913=AXIS2_PLACEMENT_3D('',#21956,#17138,#17139);
#13914=AXIS2_PLACEMENT_3D('',#21958,#17140,#17141);
#13915=AXIS2_PLACEMENT_3D('',#21960,#17142,#17143);
#13916=AXIS2_PLACEMENT_3D('',#21962,#17144,#17145);
#13917=AXIS2_PLACEMENT_3D('',#21964,#17146,#17147);
#13918=AXIS2_PLACEMENT_3D('',#21966,#17148,#17149);
#13919=AXIS2_PLACEMENT_3D('',#21968,#17150,#17151);
#13920=AXIS2_PLACEMENT_3D('',#21970,#17152,#17153);
#13921=AXIS2_PLACEMENT_3D('',#21972,#17154,#17155);
#13922=AXIS2_PLACEMENT_3D('',#21974,#17156,#17157);
#13923=AXIS2_PLACEMENT_3D('',#21976,#17158,#17159);
#13924=AXIS2_PLACEMENT_3D('',#21977,#17160,#17161);
#13925=AXIS2_PLACEMENT_3D('',#21978,#17162,#17163);
#13926=AXIS2_PLACEMENT_3D('',#21980,#17164,#17165);
#13927=AXIS2_PLACEMENT_3D('',#21982,#17167,#17168);
#13928=AXIS2_PLACEMENT_3D('',#21983,#17169,#17170);
#13929=AXIS2_PLACEMENT_3D('',#21985,#17171,#17172);
#13930=AXIS2_PLACEMENT_3D('',#21988,#17173,#17174);
#13931=AXIS2_PLACEMENT_3D('',#21990,#17175,#17176);
#13932=AXIS2_PLACEMENT_3D('',#21992,#17177,#17178);
#13933=AXIS2_PLACEMENT_3D('',#21994,#17179,#17180);
#13934=AXIS2_PLACEMENT_3D('',#21996,#17181,#17182);
#13935=AXIS2_PLACEMENT_3D('',#21998,#17183,#17184);
#13936=AXIS2_PLACEMENT_3D('',#22000,#17185,#17186);
#13937=AXIS2_PLACEMENT_3D('',#22002,#17187,#17188);
#13938=AXIS2_PLACEMENT_3D('',#22004,#17189,#17190);
#13939=AXIS2_PLACEMENT_3D('',#22006,#17191,#17192);
#13940=AXIS2_PLACEMENT_3D('',#22008,#17193,#17194);
#13941=AXIS2_PLACEMENT_3D('',#22010,#17195,#17196);
#13942=AXIS2_PLACEMENT_3D('',#22012,#17197,#17198);
#13943=AXIS2_PLACEMENT_3D('',#22014,#17199,#17200);
#13944=AXIS2_PLACEMENT_3D('',#22016,#17201,#17202);
#13945=AXIS2_PLACEMENT_3D('',#22018,#17203,#17204);
#13946=AXIS2_PLACEMENT_3D('',#22020,#17205,#17206);
#13947=AXIS2_PLACEMENT_3D('',#22022,#17207,#17208);
#13948=AXIS2_PLACEMENT_3D('',#22024,#17209,#17210);
#13949=AXIS2_PLACEMENT_3D('',#22026,#17211,#17212);
#13950=AXIS2_PLACEMENT_3D('',#22028,#17213,#17214);
#13951=AXIS2_PLACEMENT_3D('',#22030,#17215,#17216);
#13952=AXIS2_PLACEMENT_3D('',#22032,#17217,#17218);
#13953=AXIS2_PLACEMENT_3D('',#22034,#17219,#17220);
#13954=AXIS2_PLACEMENT_3D('',#22036,#17221,#17222);
#13955=AXIS2_PLACEMENT_3D('',#22038,#17223,#17224);
#13956=AXIS2_PLACEMENT_3D('',#22040,#17225,#17226);
#13957=AXIS2_PLACEMENT_3D('',#22042,#17227,#17228);
#13958=AXIS2_PLACEMENT_3D('',#22044,#17229,#17230);
#13959=AXIS2_PLACEMENT_3D('',#22046,#17231,#17232);
#13960=AXIS2_PLACEMENT_3D('',#22048,#17233,#17234);
#13961=AXIS2_PLACEMENT_3D('',#22050,#17235,#17236);
#13962=AXIS2_PLACEMENT_3D('',#22052,#17237,#17238);
#13963=AXIS2_PLACEMENT_3D('',#22054,#17239,#17240);
#13964=AXIS2_PLACEMENT_3D('',#22056,#17241,#17242);
#13965=AXIS2_PLACEMENT_3D('',#22058,#17243,#17244);
#13966=AXIS2_PLACEMENT_3D('',#22060,#17245,#17246);
#13967=AXIS2_PLACEMENT_3D('',#22062,#17247,#17248);
#13968=AXIS2_PLACEMENT_3D('',#22064,#17249,#17250);
#13969=AXIS2_PLACEMENT_3D('',#22065,#17251,#17252);
#13970=AXIS2_PLACEMENT_3D('',#22066,#17253,#17254);
#13971=AXIS2_PLACEMENT_3D('',#22068,#17255,#17256);
#13972=AXIS2_PLACEMENT_3D('',#22070,#17258,#17259);
#13973=AXIS2_PLACEMENT_3D('',#22071,#17260,#17261);
#13974=AXIS2_PLACEMENT_3D('',#22074,#17264,#17265);
#13975=AXIS2_PLACEMENT_3D('',#22076,#17267,#17268);
#13976=AXIS2_PLACEMENT_3D('',#22078,#17270,#17271);
#13977=AXIS2_PLACEMENT_3D('',#22080,#17273,#17274);
#13978=AXIS2_PLACEMENT_3D('',#22082,#17276,#17277);
#13979=AXIS2_PLACEMENT_3D('',#22084,#17279,#17280);
#13980=AXIS2_PLACEMENT_3D('',#22086,#17282,#17283);
#13981=AXIS2_PLACEMENT_3D('',#22088,#17285,#17286);
#13982=AXIS2_PLACEMENT_3D('',#22090,#17288,#17289);
#13983=AXIS2_PLACEMENT_3D('',#22092,#17291,#17292);
#13984=AXIS2_PLACEMENT_3D('',#22094,#17294,#17295);
#13985=AXIS2_PLACEMENT_3D('',#22096,#17297,#17298);
#13986=AXIS2_PLACEMENT_3D('',#22098,#17300,#17301);
#13987=AXIS2_PLACEMENT_3D('',#22100,#17303,#17304);
#13988=AXIS2_PLACEMENT_3D('',#22102,#17306,#17307);
#13989=AXIS2_PLACEMENT_3D('',#22104,#17309,#17310);
#13990=AXIS2_PLACEMENT_3D('',#22106,#17312,#17313);
#13991=AXIS2_PLACEMENT_3D('',#22108,#17315,#17316);
#13992=AXIS2_PLACEMENT_3D('',#22110,#17318,#17319);
#13993=AXIS2_PLACEMENT_3D('',#22112,#17321,#17322);
#13994=AXIS2_PLACEMENT_3D('',#22114,#17324,#17325);
#13995=AXIS2_PLACEMENT_3D('',#22116,#17327,#17328);
#13996=AXIS2_PLACEMENT_3D('',#22118,#17330,#17331);
#13997=AXIS2_PLACEMENT_3D('',#22120,#17333,#17334);
#13998=AXIS2_PLACEMENT_3D('',#22122,#17336,#17337);
#13999=AXIS2_PLACEMENT_3D('',#22124,#17339,#17340);
#14000=AXIS2_PLACEMENT_3D('',#22126,#17342,#17343);
#14001=AXIS2_PLACEMENT_3D('',#22128,#17345,#17346);
#14002=AXIS2_PLACEMENT_3D('',#22130,#17348,#17349);
#14003=AXIS2_PLACEMENT_3D('',#22132,#17351,#17352);
#14004=AXIS2_PLACEMENT_3D('',#22134,#17354,#17355);
#14005=AXIS2_PLACEMENT_3D('',#22136,#17357,#17358);
#14006=AXIS2_PLACEMENT_3D('',#22138,#17360,#17361);
#14007=AXIS2_PLACEMENT_3D('',#22140,#17363,#17364);
#14008=AXIS2_PLACEMENT_3D('',#22142,#17366,#17367);
#14009=AXIS2_PLACEMENT_3D('',#22144,#17369,#17370);
#14010=AXIS2_PLACEMENT_3D('',#22146,#17372,#17373);
#14011=AXIS2_PLACEMENT_3D('',#22148,#17375,#17376);
#14012=AXIS2_PLACEMENT_3D('',#22150,#17378,#17379);
#17046=DIRECTION('axis',(0.,0.,1.));
#17047=DIRECTION('refdir',(1.,0.,0.));
#17048=DIRECTION('center_axis',(1.,0.,6.12323399573677E-17));
#17049=DIRECTION('ref_axis',(6.12323399573677E-17,0.,-1.));
#17050=DIRECTION('',(1.,0.,6.12323399573677E-17));
#17051=DIRECTION('center_axis',(1.,0.,6.12323399573677E-17));
#17052=DIRECTION('ref_axis',(6.12323399573677E-17,0.,-1.));
#17053=DIRECTION('',(1.,0.,6.12323399573677E-17));
#17054=DIRECTION('center_axis',(0.,-1.,0.));
#17055=DIRECTION('ref_axis',(1.,0.,0.));
#17056=DIRECTION('center_axis',(0.,-1.,0.));
#17057=DIRECTION('ref_axis',(1.,0.,0.));
#17058=DIRECTION('',(0.,1.,0.));
#17059=DIRECTION('',(0.,1.,0.));
#17060=DIRECTION('center_axis',(0.,1.,0.));
#17061=DIRECTION('ref_axis',(1.,0.,0.));
#17062=DIRECTION('center_axis',(0.,0.,1.));
#17063=DIRECTION('ref_axis',(1.,0.,0.));
#17064=DIRECTION('',(0.,0.,1.));
#17065=DIRECTION('center_axis',(0.,0.,1.));
#17066=DIRECTION('ref_axis',(1.,0.,0.));
#17067=DIRECTION('',(0.,0.,1.));
#17068=DIRECTION('center_axis',(0.,1.,0.));
#17069=DIRECTION('ref_axis',(1.,0.,0.));
#17070=DIRECTION('center_axis',(0.,1.,0.));
#17071=DIRECTION('ref_axis',(1.,0.,0.));
#17072=DIRECTION('',(0.,1.,0.));
#17073=DIRECTION('',(0.,1.,0.));
#17074=DIRECTION('center_axis',(0.,-1.,0.));
#17075=DIRECTION('ref_axis',(1.,0.,0.));
#17076=DIRECTION('center_axis',(0.,1.,0.));
#17077=DIRECTION('ref_axis',(1.,0.,0.));
#17078=DIRECTION('center_axis',(0.,1.,0.));
#17079=DIRECTION('ref_axis',(1.,0.,0.));
#17080=DIRECTION('center_axis',(0.,1.,0.));
#17081=DIRECTION('ref_axis',(1.,0.,0.));
#17082=DIRECTION('center_axis',(0.,1.,0.));
#17083=DIRECTION('ref_axis',(0.951056516295154,0.,0.309016994374948));
#17084=DIRECTION('center_axis',(0.,1.,0.));
#17085=DIRECTION('ref_axis',(1.,0.,0.));
#17086=DIRECTION('center_axis',(0.,1.,0.));
#17087=DIRECTION('ref_axis',(0.809016994374947,0.,0.587785252292473));
#17088=DIRECTION('center_axis',(0.,1.,0.));
#17089=DIRECTION('ref_axis',(1.,0.,0.));
#17090=DIRECTION('center_axis',(0.,1.,0.));
#17091=DIRECTION('ref_axis',(0.587785252292473,0.,0.809016994374948));
#17092=DIRECTION('center_axis',(0.,1.,0.));
#17093=DIRECTION('ref_axis',(1.,0.,0.));
#17094=DIRECTION('center_axis',(0.,1.,0.));
#17095=DIRECTION('ref_axis',(0.309016994374947,0.,0.951056516295154));
#17096=DIRECTION('center_axis',(0.,1.,0.));
#17097=DIRECTION('ref_axis',(1.,0.,0.));
#17098=DIRECTION('center_axis',(0.,1.,0.));
#17099=DIRECTION('ref_axis',(-1.83697019872103E-16,0.,1.));
#17100=DIRECTION('center_axis',(0.,1.,0.));
#17101=DIRECTION('ref_axis',(1.,0.,0.));
#17102=DIRECTION('center_axis',(0.,1.,0.));
#17103=DIRECTION('ref_axis',(-0.309016994374948,0.,0.951056516295154));
#17104=DIRECTION('center_axis',(0.,1.,0.));
#17105=DIRECTION('ref_axis',(1.,0.,0.));
#17106=DIRECTION('center_axis',(0.,1.,0.));
#17107=DIRECTION('ref_axis',(-0.587785252292473,0.,0.809016994374947));
#17108=DIRECTION('center_axis',(0.,1.,0.));
#17109=DIRECTION('ref_axis',(1.,0.,0.));
#17110=DIRECTION('center_axis',(0.,1.,0.));
#17111=DIRECTION('ref_axis',(-0.809016994374947,0.,0.587785252292473));
#17112=DIRECTION('center_axis',(0.,1.,0.));
#17113=DIRECTION('ref_axis',(1.,0.,0.));
#17114=DIRECTION('center_axis',(0.,1.,0.));
#17115=DIRECTION('ref_axis',(-0.951056516295154,0.,0.309016994374947));
#17116=DIRECTION('center_axis',(0.,1.,0.));
#17117=DIRECTION('ref_axis',(1.,0.,0.));
#17118=DIRECTION('center_axis',(0.,1.,0.));
#17119=DIRECTION('ref_axis',(-1.,0.,-1.22464679914735E-16));
#17120=DIRECTION('center_axis',(0.,1.,0.));
#17121=DIRECTION('ref_axis',(1.,0.,0.));
#17122=DIRECTION('center_axis',(0.,1.,0.));
#17123=DIRECTION('ref_axis',(-0.951056516295154,0.,-0.309016994374948));
#17124=DIRECTION('center_axis',(0.,1.,0.));
#17125=DIRECTION('ref_axis',(1.,0.,0.));
#17126=DIRECTION('center_axis',(0.,1.,0.));
#17127=DIRECTION('ref_axis',(-0.809016994374947,0.,-0.587785252292473));
#17128=DIRECTION('center_axis',(0.,1.,0.));
#17129=DIRECTION('ref_axis',(1.,0.,0.));
#17130=DIRECTION('center_axis',(0.,1.,0.));
#17131=DIRECTION('ref_axis',(-0.587785252292473,0.,-0.809016994374948));
#17132=DIRECTION('center_axis',(0.,1.,0.));
#17133=DIRECTION('ref_axis',(1.,0.,0.));
#17134=DIRECTION('center_axis',(0.,1.,0.));
#17135=DIRECTION('ref_axis',(-0.309016994374947,0.,-0.951056516295154));
#17136=DIRECTION('center_axis',(0.,1.,0.));
#17137=DIRECTION('ref_axis',(1.,0.,0.));
#17138=DIRECTION('center_axis',(0.,1.,0.));
#17139=DIRECTION('ref_axis',(6.12323399573677E-17,0.,-1.));
#17140=DIRECTION('center_axis',(0.,1.,0.));
#17141=DIRECTION('ref_axis',(1.,0.,0.));
#17142=DIRECTION('center_axis',(0.,1.,0.));
#17143=DIRECTION('ref_axis',(0.309016994374947,0.,-0.951056516295154));
#17144=DIRECTION('center_axis',(0.,1.,0.));
#17145=DIRECTION('ref_axis',(1.,0.,0.));
#17146=DIRECTION('center_axis',(0.,1.,0.));
#17147=DIRECTION('ref_axis',(0.587785252292473,0.,-0.809016994374947));
#17148=DIRECTION('center_axis',(0.,1.,0.));
#17149=DIRECTION('ref_axis',(1.,0.,0.));
#17150=DIRECTION('center_axis',(0.,1.,0.));
#17151=DIRECTION('ref_axis',(0.809016994374947,0.,-0.587785252292473));
#17152=DIRECTION('center_axis',(0.,1.,0.));
#17153=DIRECTION('ref_axis',(1.,0.,0.));
#17154=DIRECTION('center_axis',(0.,1.,0.));
#17155=DIRECTION('ref_axis',(0.951056516295154,0.,-0.309016994374947));
#17156=DIRECTION('center_axis',(0.,1.,0.));
#17157=DIRECTION('ref_axis',(1.,0.,0.));
#17158=DIRECTION('center_axis',(0.,1.,0.));
#17159=DIRECTION('ref_axis',(1.,0.,0.));
#17160=DIRECTION('center_axis',(0.,1.,0.));
#17161=DIRECTION('ref_axis',(1.,0.,0.));
#17162=DIRECTION('center_axis',(0.,-1.,0.));
#17163=DIRECTION('ref_axis',(1.,0.,0.));
#17164=DIRECTION('center_axis',(0.,-1.,0.));
#17165=DIRECTION('ref_axis',(1.,0.,0.));
#17166=DIRECTION('',(0.,1.,0.));
#17167=DIRECTION('center_axis',(0.,1.,0.));
#17168=DIRECTION('ref_axis',(1.,0.,0.));
#17169=DIRECTION('center_axis',(0.,1.,0.));
#17170=DIRECTION('ref_axis',(1.,0.,0.));
#17171=DIRECTION('center_axis',(0.,1.,0.));
#17172=DIRECTION('ref_axis',(1.,0.,0.));
#17173=DIRECTION('center_axis',(0.,-1.,0.));
#17174=DIRECTION('ref_axis',(0.951056516295154,0.,0.309016994374948));
#17175=DIRECTION('center_axis',(0.,1.,0.));
#17176=DIRECTION('ref_axis',(1.,0.,0.));
#17177=DIRECTION('center_axis',(0.,-1.,0.));
#17178=DIRECTION('ref_axis',(1.,0.,0.));
#17179=DIRECTION('center_axis',(0.,1.,0.));
#17180=DIRECTION('ref_axis',(1.,0.,0.));
#17181=DIRECTION('center_axis',(0.,-1.,0.));
#17182=DIRECTION('ref_axis',(0.951056516295154,0.,-0.309016994374947));
#17183=DIRECTION('center_axis',(0.,1.,0.));
#17184=DIRECTION('ref_axis',(1.,0.,0.));
#17185=DIRECTION('center_axis',(0.,-1.,0.));
#17186=DIRECTION('ref_axis',(0.809016994374947,0.,-0.587785252292473));
#17187=DIRECTION('center_axis',(0.,1.,0.));
#17188=DIRECTION('ref_axis',(1.,0.,0.));
#17189=DIRECTION('center_axis',(0.,-1.,0.));
#17190=DIRECTION('ref_axis',(0.587785252292473,0.,-0.809016994374947));
#17191=DIRECTION('center_axis',(0.,1.,0.));
#17192=DIRECTION('ref_axis',(1.,0.,0.));
#17193=DIRECTION('center_axis',(0.,-1.,0.));
#17194=DIRECTION('ref_axis',(0.309016994374947,0.,-0.951056516295154));
#17195=DIRECTION('center_axis',(0.,1.,0.));
#17196=DIRECTION('ref_axis',(1.,0.,0.));
#17197=DIRECTION('center_axis',(0.,-1.,0.));
#17198=DIRECTION('ref_axis',(6.12323399573677E-17,0.,-1.));
#17199=DIRECTION('center_axis',(0.,1.,0.));
#17200=DIRECTION('ref_axis',(1.,0.,0.));
#17201=DIRECTION('center_axis',(0.,-1.,0.));
#17202=DIRECTION('ref_axis',(-0.309016994374947,0.,-0.951056516295154));
#17203=DIRECTION('center_axis',(0.,1.,0.));
#17204=DIRECTION('ref_axis',(1.,0.,0.));
#17205=DIRECTION('center_axis',(0.,-1.,0.));
#17206=DIRECTION('ref_axis',(-0.587785252292473,0.,-0.809016994374948));
#17207=DIRECTION('center_axis',(0.,1.,0.));
#17208=DIRECTION('ref_axis',(1.,0.,0.));
#17209=DIRECTION('center_axis',(0.,-1.,0.));
#17210=DIRECTION('ref_axis',(-0.809016994374947,0.,-0.587785252292473));
#17211=DIRECTION('center_axis',(0.,1.,0.));
#17212=DIRECTION('ref_axis',(1.,0.,0.));
#17213=DIRECTION('center_axis',(0.,-1.,0.));
#17214=DIRECTION('ref_axis',(-0.951056516295154,0.,-0.309016994374948));
#17215=DIRECTION('center_axis',(0.,1.,0.));
#17216=DIRECTION('ref_axis',(1.,0.,0.));
#17217=DIRECTION('center_axis',(0.,-1.,0.));
#17218=DIRECTION('ref_axis',(-1.,0.,-1.22464679914735E-16));
#17219=DIRECTION('center_axis',(0.,1.,0.));
#17220=DIRECTION('ref_axis',(1.,0.,0.));
#17221=DIRECTION('center_axis',(0.,-1.,0.));
#17222=DIRECTION('ref_axis',(-0.951056516295154,0.,0.309016994374947));
#17223=DIRECTION('center_axis',(0.,1.,0.));
#17224=DIRECTION('ref_axis',(1.,0.,0.));
#17225=DIRECTION('center_axis',(0.,-1.,0.));
#17226=DIRECTION('ref_axis',(-0.809016994374947,0.,0.587785252292473));
#17227=DIRECTION('center_axis',(0.,1.,0.));
#17228=DIRECTION('ref_axis',(1.,0.,0.));
#17229=DIRECTION('center_axis',(0.,-1.,0.));
#17230=DIRECTION('ref_axis',(-0.587785252292473,0.,0.809016994374947));
#17231=DIRECTION('center_axis',(0.,1.,0.));
#17232=DIRECTION('ref_axis',(1.,0.,0.));
#17233=DIRECTION('center_axis',(0.,-1.,0.));
#17234=DIRECTION('ref_axis',(-0.309016994374948,0.,0.951056516295154));
#17235=DIRECTION('center_axis',(0.,1.,0.));
#17236=DIRECTION('ref_axis',(1.,0.,0.));
#17237=DIRECTION('center_axis',(0.,-1.,0.));
#17238=DIRECTION('ref_axis',(-1.83697019872103E-16,0.,1.));
#17239=DIRECTION('center_axis',(0.,1.,0.));
#17240=DIRECTION('ref_axis',(1.,0.,0.));
#17241=DIRECTION('center_axis',(0.,-1.,0.));
#17242=DIRECTION('ref_axis',(0.309016994374947,0.,0.951056516295154));
#17243=DIRECTION('center_axis',(0.,1.,0.));
#17244=DIRECTION('ref_axis',(1.,0.,0.));
#17245=DIRECTION('center_axis',(0.,-1.,0.));
#17246=DIRECTION('ref_axis',(0.587785252292473,0.,0.809016994374948));
#17247=DIRECTION('center_axis',(0.,1.,0.));
#17248=DIRECTION('ref_axis',(1.,0.,0.));
#17249=DIRECTION('center_axis',(0.,-1.,0.));
#17250=DIRECTION('ref_axis',(0.809016994374947,0.,0.587785252292473));
#17251=DIRECTION('center_axis',(0.,1.,0.));
#17252=DIRECTION('ref_axis',(1.,0.,0.));
#17253=DIRECTION('center_axis',(0.,1.,0.));
#17254=DIRECTION('ref_axis',(1.,0.,0.));
#17255=DIRECTION('center_axis',(0.,1.,0.));
#17256=DIRECTION('ref_axis',(1.,0.,0.));
#17257=DIRECTION('',(0.,-1.,0.));
#17258=DIRECTION('center_axis',(0.,1.,0.));
#17259=DIRECTION('ref_axis',(1.,0.,0.));
#17260=DIRECTION('center_axis',(0.,1.,0.));
#17261=DIRECTION('ref_axis',(-0.951056516295153,0.,-0.309016994374948));
#17262=DIRECTION('',(0.,-1.,0.));
#17263=DIRECTION('',(0.,1.,0.));
#17264=DIRECTION('center_axis',(0.,1.,0.));
#17265=DIRECTION('ref_axis',(1.,0.,0.));
#17266=DIRECTION('',(0.,-1.,0.));
#17267=DIRECTION('center_axis',(0.,1.,0.));
#17268=DIRECTION('ref_axis',(-0.809016994374947,0.,-0.587785252292473));
#17269=DIRECTION('',(0.,1.,0.));
#17270=DIRECTION('center_axis',(0.,1.,0.));
#17271=DIRECTION('ref_axis',(1.,0.,0.));
#17272=DIRECTION('',(0.,-1.,0.));
#17273=DIRECTION('center_axis',(0.,1.,0.));
#17274=DIRECTION('ref_axis',(-0.587785252292473,0.,-0.809016994374947));
#17275=DIRECTION('',(0.,1.,0.));
#17276=DIRECTION('center_axis',(0.,1.,0.));
#17277=DIRECTION('ref_axis',(1.,0.,0.));
#17278=DIRECTION('',(0.,-1.,0.));
#17279=DIRECTION('center_axis',(0.,1.,0.));
#17280=DIRECTION('ref_axis',(-0.309016994374947,0.,-0.951056516295154));
#17281=DIRECTION('',(0.,1.,0.));
#17282=DIRECTION('center_axis',(0.,1.,0.));
#17283=DIRECTION('ref_axis',(1.,0.,0.));
#17284=DIRECTION('',(0.,-1.,0.));
#17285=DIRECTION('center_axis',(0.,1.,0.));
#17286=DIRECTION('ref_axis',(-1.37927510063224E-16,0.,-1.));
#17287=DIRECTION('',(0.,1.,0.));
#17288=DIRECTION('center_axis',(0.,1.,0.));
#17289=DIRECTION('ref_axis',(1.,0.,0.));
#17290=DIRECTION('',(0.,-1.,0.));
#17291=DIRECTION('center_axis',(0.,1.,0.));
#17292=DIRECTION('ref_axis',(0.309016994374948,0.,-0.951056516295154));
#17293=DIRECTION('',(0.,1.,0.));
#17294=DIRECTION('center_axis',(0.,1.,0.));
#17295=DIRECTION('ref_axis',(1.,0.,0.));
#17296=DIRECTION('',(0.,-1.,0.));
#17297=DIRECTION('center_axis',(0.,1.,0.));
#17298=DIRECTION('ref_axis',(0.587785252292473,0.,-0.809016994374948));
#17299=DIRECTION('',(0.,1.,0.));
#17300=DIRECTION('center_axis',(0.,1.,0.));
#17301=DIRECTION('ref_axis',(1.,0.,0.));
#17302=DIRECTION('',(0.,-1.,0.));
#17303=DIRECTION('center_axis',(0.,1.,0.));
#17304=DIRECTION('ref_axis',(0.809016994374948,0.,-0.587785252292473));
#17305=DIRECTION('',(0.,1.,0.));
#17306=DIRECTION('center_axis',(0.,1.,0.));
#17307=DIRECTION('ref_axis',(1.,0.,0.));
#17308=DIRECTION('',(0.,-1.,0.));
#17309=DIRECTION('center_axis',(0.,1.,0.));
#17310=DIRECTION('ref_axis',(0.951056516295154,0.,-0.309016994374947));
#17311=DIRECTION('',(0.,1.,0.));
#17312=DIRECTION('center_axis',(0.,1.,0.));
#17313=DIRECTION('ref_axis',(1.,0.,0.));
#17314=DIRECTION('',(0.,-1.,0.));
#17315=DIRECTION('center_axis',(0.,1.,0.));
#17316=DIRECTION('ref_axis',(1.,0.,-1.99159850020592E-16));
#17317=DIRECTION('',(0.,1.,0.));
#17318=DIRECTION('center_axis',(0.,1.,0.));
#17319=DIRECTION('ref_axis',(1.,0.,0.));
#17320=DIRECTION('',(0.,-1.,0.));
#17321=DIRECTION('center_axis',(0.,1.,0.));
#17322=DIRECTION('ref_axis',(0.951056516295154,0.,0.309016994374948));
#17323=DIRECTION('',(0.,1.,0.));
#17324=DIRECTION('center_axis',(0.,1.,0.));
#17325=DIRECTION('ref_axis',(1.,0.,0.));
#17326=DIRECTION('',(0.,-1.,0.));
#17327=DIRECTION('center_axis',(0.,1.,0.));
#17328=DIRECTION('ref_axis',(0.809016994374948,0.,0.587785252292473));
#17329=DIRECTION('',(0.,1.,0.));
#17330=DIRECTION('center_axis',(0.,1.,0.));
#17331=DIRECTION('ref_axis',(1.,0.,0.));
#17332=DIRECTION('',(0.,-1.,0.));
#17333=DIRECTION('center_axis',(0.,1.,0.));
#17334=DIRECTION('ref_axis',(0.587785252292473,0.,0.809016994374948));
#17335=DIRECTION('',(0.,1.,0.));
#17336=DIRECTION('center_axis',(0.,1.,0.));
#17337=DIRECTION('ref_axis',(1.,0.,0.));
#17338=DIRECTION('',(0.,-1.,0.));
#17339=DIRECTION('center_axis',(0.,1.,0.));
#17340=DIRECTION('ref_axis',(0.309016994374947,0.,0.951056516295154));
#17341=DIRECTION('',(0.,1.,0.));
#17342=DIRECTION('center_axis',(0.,1.,0.));
#17343=DIRECTION('ref_axis',(1.,0.,0.));
#17344=DIRECTION('',(0.,-1.,0.));
#17345=DIRECTION('center_axis',(0.,1.,0.));
#17346=DIRECTION('ref_axis',(2.6039218997796E-16,0.,1.));
#17347=DIRECTION('',(0.,1.,0.));
#17348=DIRECTION('center_axis',(0.,1.,0.));
#17349=DIRECTION('ref_axis',(1.,0.,0.));
#17350=DIRECTION('',(0.,-1.,0.));
#17351=DIRECTION('center_axis',(0.,1.,0.));
#17352=DIRECTION('ref_axis',(-0.309016994374948,0.,0.951056516295153));
#17353=DIRECTION('',(0.,1.,0.));
#17354=DIRECTION('center_axis',(0.,1.,0.));
#17355=DIRECTION('ref_axis',(1.,0.,0.));
#17356=DIRECTION('',(0.,-1.,0.));
#17357=DIRECTION('center_axis',(0.,1.,0.));
#17358=DIRECTION('ref_axis',(-0.587785252292474,0.,0.809016994374947));
#17359=DIRECTION('',(0.,1.,0.));
#17360=DIRECTION('center_axis',(0.,1.,0.));
#17361=DIRECTION('ref_axis',(1.,0.,0.));
#17362=DIRECTION('',(0.,-1.,0.));
#17363=DIRECTION('center_axis',(0.,1.,0.));
#17364=DIRECTION('ref_axis',(-0.809016994374948,0.,0.587785252292473));
#17365=DIRECTION('',(0.,1.,0.));
#17366=DIRECTION('center_axis',(0.,1.,0.));
#17367=DIRECTION('ref_axis',(1.,0.,0.));
#17368=DIRECTION('',(0.,-1.,0.));
#17369=DIRECTION('center_axis',(0.,1.,0.));
#17370=DIRECTION('ref_axis',(-0.951056516295154,0.,0.309016994374948));
#17371=DIRECTION('',(0.,1.,0.));
#17372=DIRECTION('center_axis',(0.,1.,0.));
#17373=DIRECTION('ref_axis',(1.,0.,0.));
#17374=DIRECTION('',(0.,1.,0.));
#17375=DIRECTION('center_axis',(0.,1.,0.));
#17376=DIRECTION('ref_axis',(-1.,0.,-1.22464679914735E-16));
#17377=DIRECTION('',(0.,-1.,0.));
#17378=DIRECTION('center_axis',(0.,1.,0.));
#17379=DIRECTION('ref_axis',(1.,0.,0.));
#21549=CARTESIAN_POINT('',(0.,0.,0.));
#21550=CARTESIAN_POINT('Origin',(0.,-0.45,0.));
#21551=CARTESIAN_POINT('',(-0.65,-0.325,-3.9801020972289E-17));
#21552=CARTESIAN_POINT('',(-0.637867541108654,-0.45,0.125));
#21553=CARTESIAN_POINT('Ctrl Pts',(-0.65,-0.325,-6.93889390390723E-17));
#21554=CARTESIAN_POINT('Ctrl Pts',(-0.65,-0.325,0.0157371373481997));
#21555=CARTESIAN_POINT('Ctrl Pts',(-0.649370620646074,-0.328153081062251,
0.0324967135411163));
#21556=CARTESIAN_POINT('Ctrl Pts',(-0.647096224417991,-0.340922081922822,
0.0632828231545122));
#21557=CARTESIAN_POINT('Ctrl Pts',(-0.645482573914132,-0.350535859112198,
0.0773125544088347));
#21558=CARTESIAN_POINT('Ctrl Pts',(-0.642442040715078,-0.372687974598127,
0.0994646698947638));
#21559=CARTESIAN_POINT('Ctrl Pts',(-0.640815160902589,-0.386717480603274,
0.109078032552995));
#21560=CARTESIAN_POINT('Ctrl Pts',(-0.63851034608138,-0.417502809542363,
0.121846732641678));
#21561=CARTESIAN_POINT('Ctrl Pts',(-0.637867541108654,-0.434262111007648,
0.125));
#21562=CARTESIAN_POINT('Ctrl Pts',(-0.637867541108654,-0.45,0.125));
#21563=CARTESIAN_POINT('',(-0.65,-0.575,-3.9801020972289E-17));
#21564=CARTESIAN_POINT('Ctrl Pts',(-0.65,-0.575,-3.46944695195361E-18));
#21565=CARTESIAN_POINT('Ctrl Pts',(-0.65,-0.575,-0.0157371373481998));
#21566=CARTESIAN_POINT('Ctrl Pts',(-0.649370620646074,-0.571846918937749,
-0.0324967135411164));
#21567=CARTESIAN_POINT('Ctrl Pts',(-0.647096224417991,-0.559077918077178,
-0.0632828231545123));
#21568=CARTESIAN_POINT('Ctrl Pts',(-0.645482573914132,-0.549464140887802,
-0.0773125544088349));
#21569=CARTESIAN_POINT('Ctrl Pts',(-0.642442040715078,-0.527312025401873,
-0.099464669894764));
#21570=CARTESIAN_POINT('Ctrl Pts',(-0.640815160902589,-0.513282519396725,
-0.109078032552995));
#21571=CARTESIAN_POINT('Ctrl Pts',(-0.63851034608138,-0.482497190457637,
-0.121846732641678));
#21572=CARTESIAN_POINT('Ctrl Pts',(-0.637867541108654,-0.465737888992352,
-0.125));
#21573=CARTESIAN_POINT('Ctrl Pts',(-0.637867541108654,-0.434262111007648,
-0.125));
#21574=CARTESIAN_POINT('Ctrl Pts',(-0.63851034608138,-0.417502809542363,
-0.121846732641678));
#21575=CARTESIAN_POINT('Ctrl Pts',(-0.640815160902589,-0.386717480603275,
-0.109078032552995));
#21576=CARTESIAN_POINT('Ctrl Pts',(-0.642442040715078,-0.372687974598127,
-0.099464669894764));
#21577=CARTESIAN_POINT('Ctrl Pts',(-0.645482573914132,-0.350535859112198,
-0.077312554408835));
#21578=CARTESIAN_POINT('Ctrl Pts',(-0.647096224417991,-0.340922081922822,
-0.0632828231545124));
#21579=CARTESIAN_POINT('Ctrl Pts',(-0.649370620646074,-0.328153081062251,
-0.0324967135411165));
#21580=CARTESIAN_POINT('Ctrl Pts',(-0.65,-0.325,-0.0157371373481999));
#21581=CARTESIAN_POINT('Ctrl Pts',(-0.65,-0.325,-8.32667268468867E-17));
#21582=CARTESIAN_POINT('Ctrl Pts',(-0.637867541108654,-0.45,0.125));
#21583=CARTESIAN_POINT('Ctrl Pts',(-0.637867541108654,-0.465737888992352,
0.125));
#21584=CARTESIAN_POINT('Ctrl Pts',(-0.63851034608138,-0.482497190457637,
0.121846732641678));
#21585=CARTESIAN_POINT('Ctrl Pts',(-0.640815160902589,-0.513282519396725,
0.109078032552995));
#21586=CARTESIAN_POINT('Ctrl Pts',(-0.642442040715078,-0.527312025401873,
0.0994646698947639));
#21587=CARTESIAN_POINT('Ctrl Pts',(-0.645482573914132,-0.549464140887802,
0.0773125544088349));
#21588=CARTESIAN_POINT('Ctrl Pts',(-0.647096224417991,-0.559077918077178,
0.0632828231545123));
#21589=CARTESIAN_POINT('Ctrl Pts',(-0.649370620646074,-0.571846918937749,
0.0324967135411164));
#21590=CARTESIAN_POINT('Ctrl Pts',(-0.65,-0.575,0.0157371373481998));
#21591=CARTESIAN_POINT('Ctrl Pts',(-0.65,-0.575,-2.08166817117217E-17));
#21592=CARTESIAN_POINT('',(-0.379967103839267,-0.45,0.125));
#21593=CARTESIAN_POINT('',(-7.65404249467096E-18,-0.45,0.125));
#21594=CARTESIAN_POINT('',(-0.4,-0.575,5.41097774720219E-18));
#21595=CARTESIAN_POINT('Ctrl Pts',(-0.4,-0.575,-3.81639164714898E-17));
#21596=CARTESIAN_POINT('Ctrl Pts',(-0.4,-0.575,0.0158075115832675));
#21597=CARTESIAN_POINT('Ctrl Pts',(-0.398970551469948,-0.571819306519379,
0.0325978607437828));
#21598=CARTESIAN_POINT('Ctrl Pts',(-0.395252954914593,-0.559029081159106,
0.0633657881355917));
#21599=CARTESIAN_POINT('Ctrl Pts',(-0.392612801026882,-0.549425200318011,
0.0773514949786256));
#21600=CARTESIAN_POINT('Ctrl Pts',(-0.38761064154154,-0.527347592689753,
0.0994291026068839));
#21601=CARTESIAN_POINT('Ctrl Pts',(-0.384911758361269,-0.51336346023721,
0.109029967924066));
#21602=CARTESIAN_POINT('Ctrl Pts',(-0.381057715344782,-0.48260129709332,
0.121817958968287));
#21603=CARTESIAN_POINT('Ctrl Pts',(-0.379967103839267,-0.465813100629203,
0.125));
#21604=CARTESIAN_POINT('Ctrl Pts',(-0.379967103839267,-0.45,0.125));
#21605=CARTESIAN_POINT('',(-0.379967103839267,-0.45,-0.125));
#21606=CARTESIAN_POINT('Ctrl Pts',(-0.379967103839267,-0.45,-0.125));
#21607=CARTESIAN_POINT('Ctrl Pts',(-0.379967103839267,-0.465813100629203,
-0.125));
#21608=CARTESIAN_POINT('Ctrl Pts',(-0.381057715344782,-0.48260129709332,
-0.121817958968287));
#21609=CARTESIAN_POINT('Ctrl Pts',(-0.384911758361269,-0.51336346023721,
-0.109029967924066));
#21610=CARTESIAN_POINT('Ctrl Pts',(-0.38761064154154,-0.527347592689753,
-0.099429102606884));
#21611=CARTESIAN_POINT('Ctrl Pts',(-0.392612801026882,-0.549425200318011,
-0.0773514949786257));
#21612=CARTESIAN_POINT('Ctrl Pts',(-0.395252954914593,-0.559029081159106,
-0.0633657881355918));
#21613=CARTESIAN_POINT('Ctrl Pts',(-0.398970551469948,-0.571819306519379,
-0.0325978607437828));
#21614=CARTESIAN_POINT('Ctrl Pts',(-0.4,-0.575,-0.0158075115832676));
#21615=CARTESIAN_POINT('Ctrl Pts',(-0.4,-0.575,-4.16333634234434E-17));
#21616=CARTESIAN_POINT('',(-0.4,-0.325,2.96971064108775E-17));
#21617=CARTESIAN_POINT('Ctrl Pts',(-0.4,-0.325,1.04083408558608E-17));
#21618=CARTESIAN_POINT('Ctrl Pts',(-0.4,-0.325,-0.0158075115832676));
#21619=CARTESIAN_POINT('Ctrl Pts',(-0.398970551469948,-0.328180693480621,
-0.0325978607437828));
#21620=CARTESIAN_POINT('Ctrl Pts',(-0.395252954914593,-0.340970918840894,
-0.0633657881355918));
#21621=CARTESIAN_POINT('Ctrl Pts',(-0.392612801026882,-0.350574799681989,
-0.0773514949786256));
#21622=CARTESIAN_POINT('Ctrl Pts',(-0.38761064154154,-0.372652407310247,
-0.0994291026068839));
#21623=CARTESIAN_POINT('Ctrl Pts',(-0.384911758361269,-0.38663653976279,
-0.109029967924066));
#21624=CARTESIAN_POINT('Ctrl Pts',(-0.381057715344782,-0.41739870290668,
-0.121817958968287));
#21625=CARTESIAN_POINT('Ctrl Pts',(-0.379967103839267,-0.434186899370797,
-0.125));
#21626=CARTESIAN_POINT('Ctrl Pts',(-0.379967103839267,-0.45,-0.125));
#21627=CARTESIAN_POINT('Ctrl Pts',(-0.379967103839267,-0.45,0.125));
#21628=CARTESIAN_POINT('Ctrl Pts',(-0.379967103839267,-0.434186899370797,
0.125));
#21629=CARTESIAN_POINT('Ctrl Pts',(-0.381057715344782,-0.41739870290668,
0.121817958968287));
#21630=CARTESIAN_POINT('Ctrl Pts',(-0.384911758361269,-0.38663653976279,
0.109029967924066));
#21631=CARTESIAN_POINT('Ctrl Pts',(-0.38761064154154,-0.372652407310247,
0.0994291026068839));
#21632=CARTESIAN_POINT('Ctrl Pts',(-0.392612801026882,-0.350574799681989,
0.0773514949786257));
#21633=CARTESIAN_POINT('Ctrl Pts',(-0.395252954914593,-0.340970918840894,
0.0633657881355918));
#21634=CARTESIAN_POINT('Ctrl Pts',(-0.398970551469948,-0.328180693480621,
0.0325978607437829));
#21635=CARTESIAN_POINT('Ctrl Pts',(-0.4,-0.325,0.0158075115832676));
#21636=CARTESIAN_POINT('Ctrl Pts',(-0.4,-0.325,1.38777878078145E-17));
#21637=CARTESIAN_POINT('Origin',(0.,-0.45,0.));
#21638=CARTESIAN_POINT('',(0.379967103839267,-0.45,-0.125));
#21639=CARTESIAN_POINT('',(0.379967103839267,-0.45,0.125));
#21640=CARTESIAN_POINT('Ctrl Pts',(0.379967103839267,-0.45,-0.125));
#21641=CARTESIAN_POINT('Ctrl Pts',(0.379967103839267,-0.434186899370797,
-0.125));
#21642=CARTESIAN_POINT('Ctrl Pts',(0.381057715344782,-0.41739870290668,
-0.121817958968287));
#21643=CARTESIAN_POINT('Ctrl Pts',(0.384911758361269,-0.38663653976279,
-0.109029967924066));
#21644=CARTESIAN_POINT('Ctrl Pts',(0.38761064154154,-0.372652407310247,
-0.0994291026068839));
#21645=CARTESIAN_POINT('Ctrl Pts',(0.392612801026882,-0.350574799681989,
-0.0773514949786256));
#21646=CARTESIAN_POINT('Ctrl Pts',(0.395252954914593,-0.340970918840894,
-0.0633657881355917));
#21647=CARTESIAN_POINT('Ctrl Pts',(0.398970551469948,-0.328180693480621,
-0.0325978607437828));
#21648=CARTESIAN_POINT('Ctrl Pts',(0.4,-0.325,-0.0158075115832675));
#21649=CARTESIAN_POINT('Ctrl Pts',(0.4,-0.325,0.0158075115832676));
#21650=CARTESIAN_POINT('Ctrl Pts',(0.398970551469948,-0.328180693480621,
0.0325978607437829));
#21651=CARTESIAN_POINT('Ctrl Pts',(0.395252954914593,-0.340970918840894,
0.0633657881355918));
#21652=CARTESIAN_POINT('Ctrl Pts',(0.392612801026882,-0.350574799681989,
0.0773514949786257));
#21653=CARTESIAN_POINT('Ctrl Pts',(0.38761064154154,-0.372652407310247,
0.099429102606884));
#21654=CARTESIAN_POINT('Ctrl Pts',(0.384911758361269,-0.38663653976279,
0.109029967924066));
#21655=CARTESIAN_POINT('Ctrl Pts',(0.381057715344782,-0.41739870290668,
0.121817958968287));
#21656=CARTESIAN_POINT('Ctrl Pts',(0.379967103839267,-0.434186899370797,
0.125));
#21657=CARTESIAN_POINT('Ctrl Pts',(0.379967103839267,-0.45,0.125));
#21658=CARTESIAN_POINT('Ctrl Pts',(0.379967103839267,-0.45,0.125));
#21659=CARTESIAN_POINT('Ctrl Pts',(0.379967103839267,-0.465813100629203,
0.125));
#21660=CARTESIAN_POINT('Ctrl Pts',(0.381057715344782,-0.48260129709332,
0.121817958968287));
#21661=CARTESIAN_POINT('Ctrl Pts',(0.384911758361269,-0.51336346023721,
0.109029967924066));
#21662=CARTESIAN_POINT('Ctrl Pts',(0.38761064154154,-0.527347592689753,
0.0994291026068839));
#21663=CARTESIAN_POINT('Ctrl Pts',(0.392612801026882,-0.549425200318011,
0.0773514949786257));
#21664=CARTESIAN_POINT('Ctrl Pts',(0.395252954914593,-0.559029081159106,
0.0633657881355918));
#21665=CARTESIAN_POINT('Ctrl Pts',(0.398970551469948,-0.571819306519379,
0.0325978607437829));
#21666=CARTESIAN_POINT('Ctrl Pts',(0.4,-0.575,0.0158075115832676));
#21667=CARTESIAN_POINT('Ctrl Pts',(0.4,-0.575,-0.0158075115832676));
#21668=CARTESIAN_POINT('Ctrl Pts',(0.398970551469948,-0.57181930651938,
-0.0325978607437828));
#21669=CARTESIAN_POINT('Ctrl Pts',(0.395252954914593,-0.559029081159106,
-0.0633657881355918));
#21670=CARTESIAN_POINT('Ctrl Pts',(0.392612801026882,-0.549425200318011,
-0.0773514949786257));
#21671=CARTESIAN_POINT('Ctrl Pts',(0.38761064154154,-0.527347592689753,
-0.0994291026068839));
#21672=CARTESIAN_POINT('Ctrl Pts',(0.384911758361269,-0.51336346023721,
-0.109029967924066));
#21673=CARTESIAN_POINT('Ctrl Pts',(0.381057715344782,-0.48260129709332,
-0.121817958968287));
#21674=CARTESIAN_POINT('Ctrl Pts',(0.379967103839267,-0.465813100629203,
-0.125));
#21675=CARTESIAN_POINT('Ctrl Pts',(0.379967103839267,-0.45,-0.125));
#21676=CARTESIAN_POINT('',(0.637867541108654,-0.45,0.125));
#21677=CARTESIAN_POINT('',(-7.65404249467096E-18,-0.45,0.125));
#21678=CARTESIAN_POINT('',(0.65,-0.575,3.9801020972289E-17));
#21679=CARTESIAN_POINT('Ctrl Pts',(0.65,-0.575,5.55111512312578E-17));
#21680=CARTESIAN_POINT('Ctrl Pts',(0.65,-0.575,0.0157371373481999));
#21681=CARTESIAN_POINT('Ctrl Pts',(0.649370620646074,-0.571846918937749,
0.0324967135411165));
#21682=CARTESIAN_POINT('Ctrl Pts',(0.647096224417991,-0.559077918077178,
0.0632828231545124));
#21683=CARTESIAN_POINT('Ctrl Pts',(0.645482573914132,-0.549464140887802,
0.077312554408835));
#21684=CARTESIAN_POINT('Ctrl Pts',(0.642442040715078,-0.527312025401873,
0.099464669894764));
#21685=CARTESIAN_POINT('Ctrl Pts',(0.640815160902589,-0.513282519396725,
0.109078032552995));
#21686=CARTESIAN_POINT('Ctrl Pts',(0.63851034608138,-0.482497190457637,
0.121846732641678));
#21687=CARTESIAN_POINT('Ctrl Pts',(0.637867541108654,-0.465737888992352,
0.125));
#21688=CARTESIAN_POINT('Ctrl Pts',(0.637867541108654,-0.45,0.125));
#21689=CARTESIAN_POINT('',(0.65,-0.325,3.9801020972289E-17));
#21690=CARTESIAN_POINT('Ctrl Pts',(0.65,-0.325,6.93889390390723E-18));
#21691=CARTESIAN_POINT('Ctrl Pts',(0.65,-0.325,-0.0157371373481998));
#21692=CARTESIAN_POINT('Ctrl Pts',(0.649370620646074,-0.328153081062251,
-0.0324967135411164));
#21693=CARTESIAN_POINT('Ctrl Pts',(0.647096224417991,-0.340922081922822,
-0.0632828231545123));
#21694=CARTESIAN_POINT('Ctrl Pts',(0.645482573914132,-0.350535859112198,
-0.0773125544088349));
#21695=CARTESIAN_POINT('Ctrl Pts',(0.642442040715078,-0.372687974598127,
-0.0994646698947639));
#21696=CARTESIAN_POINT('Ctrl Pts',(0.640815160902588,-0.386717480603275,
-0.109078032552995));
#21697=CARTESIAN_POINT('Ctrl Pts',(0.63851034608138,-0.417502809542363,
-0.121846732641678));
#21698=CARTESIAN_POINT('Ctrl Pts',(0.637867541108654,-0.434262111007648,
-0.125));
#21699=CARTESIAN_POINT('Ctrl Pts',(0.637867541108654,-0.465737888992352,
-0.125));
#21700=CARTESIAN_POINT('Ctrl Pts',(0.63851034608138,-0.482497190457637,
-0.121846732641678));
#21701=CARTESIAN_POINT('Ctrl Pts',(0.640815160902589,-0.513282519396725,
-0.109078032552995));
#21702=CARTESIAN_POINT('Ctrl Pts',(0.642442040715078,-0.527312025401873,
-0.0994646698947639));
#21703=CARTESIAN_POINT('Ctrl Pts',(0.645482573914132,-0.549464140887802,
-0.0773125544088348));
#21704=CARTESIAN_POINT('Ctrl Pts',(0.647096224417991,-0.559077918077178,
-0.0632828231545123));
#21705=CARTESIAN_POINT('Ctrl Pts',(0.649370620646074,-0.571846918937749,
-0.0324967135411164));
#21706=CARTESIAN_POINT('Ctrl Pts',(0.65,-0.575,-0.0157371373481998));
#21707=CARTESIAN_POINT('Ctrl Pts',(0.65,-0.575,6.24500451351651E-17));
#21708=CARTESIAN_POINT('Ctrl Pts',(0.637867541108654,-0.45,0.125));
#21709=CARTESIAN_POINT('Ctrl Pts',(0.637867541108654,-0.434262111007648,
0.125));
#21710=CARTESIAN_POINT('Ctrl Pts',(0.63851034608138,-0.417502809542363,
0.121846732641678));
#21711=CARTESIAN_POINT('Ctrl Pts',(0.640815160902589,-0.386717480603274,
0.109078032552995));
#21712=CARTESIAN_POINT('Ctrl Pts',(0.642442040715078,-0.372687974598127,
0.0994646698947639));
#21713=CARTESIAN_POINT('Ctrl Pts',(0.645482573914132,-0.350535859112198,
0.0773125544088348));
#21714=CARTESIAN_POINT('Ctrl Pts',(0.647096224417991,-0.340922081922822,
0.0632828231545123));
#21715=CARTESIAN_POINT('Ctrl Pts',(0.649370620646074,-0.328153081062251,
0.0324967135411164));
#21716=CARTESIAN_POINT('Ctrl Pts',(0.65,-0.325,0.0157371373481998));
#21717=CARTESIAN_POINT('Ctrl Pts',(0.65,-0.325,-6.93889390390723E-18));
#21718=CARTESIAN_POINT('Origin',(0.,-0.1,0.));
#21719=CARTESIAN_POINT('',(-0.65,-0.8,7.9602041944578E-17));
#21720=CARTESIAN_POINT('Origin',(0.,-0.8,0.));
#21721=CARTESIAN_POINT('',(-0.65,-0.1,-7.9602041944578E-17));
#21722=CARTESIAN_POINT('',(-0.65,-0.1,7.9602041944578E-17));
#21723=CARTESIAN_POINT('',(-0.65,-0.1,-7.9602041944578E-17));
#21724=CARTESIAN_POINT('Origin',(0.,-0.1,0.));
#21725=CARTESIAN_POINT('',(0.,-0.575,-0.65));
#21726=CARTESIAN_POINT('',(0.,-0.325,-0.65));
#21727=CARTESIAN_POINT('Ctrl Pts',(-1.73472347597681E-17,-0.575,-0.65));
#21728=CARTESIAN_POINT('Ctrl Pts',(0.0157371373481998,-0.575,-0.65));
#21729=CARTESIAN_POINT('Ctrl Pts',(0.0324967135411164,-0.571846918937749,
-0.649370620646074));
#21730=CARTESIAN_POINT('Ctrl Pts',(0.0632828231545123,-0.559077918077178,
-0.647096224417991));
#21731=CARTESIAN_POINT('Ctrl Pts',(0.0773125544088349,-0.549464140887802,
-0.645482573914132));
#21732=CARTESIAN_POINT('Ctrl Pts',(0.099464669894764,-0.527312025401873,
-0.642442040715078));
#21733=CARTESIAN_POINT('Ctrl Pts',(0.109078032552995,-0.513282519396725,
-0.640815160902589));
#21734=CARTESIAN_POINT('Ctrl Pts',(0.121846732641678,-0.482497190457636,
-0.63851034608138));
#21735=CARTESIAN_POINT('Ctrl Pts',(0.125,-0.465737888992352,-0.637867541108654));
#21736=CARTESIAN_POINT('Ctrl Pts',(0.125,-0.434262111007648,-0.637867541108654));
#21737=CARTESIAN_POINT('Ctrl Pts',(0.121846732641678,-0.417502809542364,
-0.63851034608138));
#21738=CARTESIAN_POINT('Ctrl Pts',(0.109078032552995,-0.386717480603275,
-0.640815160902589));
#21739=CARTESIAN_POINT('Ctrl Pts',(0.099464669894764,-0.372687974598127,
-0.642442040715078));
#21740=CARTESIAN_POINT('Ctrl Pts',(0.0773125544088349,-0.350535859112198,
-0.645482573914132));
#21741=CARTESIAN_POINT('Ctrl Pts',(0.0632828231545123,-0.340922081922822,
-0.647096224417991));
#21742=CARTESIAN_POINT('Ctrl Pts',(0.0324967135411164,-0.328153081062251,
-0.649370620646074));
#21743=CARTESIAN_POINT('Ctrl Pts',(0.0157371373481999,-0.325,-0.65));
#21744=CARTESIAN_POINT('Ctrl Pts',(4.5102810375397E-17,-0.325,-0.65));
#21745=CARTESIAN_POINT('',(-0.125,-0.45,-0.637867541108654));
#21746=CARTESIAN_POINT('Ctrl Pts',(4.85722573273506E-17,-0.325,-0.65));
#21747=CARTESIAN_POINT('Ctrl Pts',(-0.0157371373481997,-0.325,-0.65));
#21748=CARTESIAN_POINT('Ctrl Pts',(-0.0324967135411163,-0.328153081062251,
-0.649370620646074));
#21749=CARTESIAN_POINT('Ctrl Pts',(-0.0632828231545122,-0.340922081922822,
-0.647096224417991));
#21750=CARTESIAN_POINT('Ctrl Pts',(-0.0773125544088348,-0.350535859112198,
-0.645482573914132));
#21751=CARTESIAN_POINT('Ctrl Pts',(-0.0994646698947639,-0.372687974598127,
-0.642442040715078));
#21752=CARTESIAN_POINT('Ctrl Pts',(-0.109078032552995,-0.386717480603274,
-0.640815160902589));
#21753=CARTESIAN_POINT('Ctrl Pts',(-0.121846732641678,-0.417502809542363,
-0.63851034608138));
#21754=CARTESIAN_POINT('Ctrl Pts',(-0.125,-0.434262111007648,-0.637867541108654));
#21755=CARTESIAN_POINT('Ctrl Pts',(-0.125,-0.45,-0.637867541108654));
#21756=CARTESIAN_POINT('Ctrl Pts',(-0.125,-0.45,-0.637867541108654));
#21757=CARTESIAN_POINT('Ctrl Pts',(-0.125,-0.465737888992352,-0.637867541108654));
#21758=CARTESIAN_POINT('Ctrl Pts',(-0.121846732641678,-0.482497190457636,
-0.63851034608138));
#21759=CARTESIAN_POINT('Ctrl Pts',(-0.109078032552995,-0.513282519396725,
-0.640815160902589));
#21760=CARTESIAN_POINT('Ctrl Pts',(-0.099464669894764,-0.527312025401873,
-0.642442040715078));
#21761=CARTESIAN_POINT('Ctrl Pts',(-0.0773125544088349,-0.549464140887802,
-0.645482573914132));
#21762=CARTESIAN_POINT('Ctrl Pts',(-0.0632828231545124,-0.559077918077178,
-0.647096224417991));
#21763=CARTESIAN_POINT('Ctrl Pts',(-0.0324967135411165,-0.571846918937749,
-0.649370620646074));
#21764=CARTESIAN_POINT('Ctrl Pts',(-0.0157371373481998,-0.575,-0.65));
#21765=CARTESIAN_POINT('Ctrl Pts',(-1.73472347597681E-17,-0.575,-0.65));
#21766=CARTESIAN_POINT('',(0.,-0.325,0.65));
#21767=CARTESIAN_POINT('',(0.,-0.575,0.65));
#21768=CARTESIAN_POINT('Ctrl Pts',(2.77555756156289E-17,-0.325,0.65));
#21769=CARTESIAN_POINT('Ctrl Pts',(0.0157371373481998,-0.325,0.65));
#21770=CARTESIAN_POINT('Ctrl Pts',(0.0324967135411164,-0.328153081062251,
0.649370620646074));
#21771=CARTESIAN_POINT('Ctrl Pts',(0.0632828231545123,-0.340922081922822,
0.647096224417991));
#21772=CARTESIAN_POINT('Ctrl Pts',(0.0773125544088349,-0.350535859112198,
0.645482573914132));
#21773=CARTESIAN_POINT('Ctrl Pts',(0.099464669894764,-0.372687974598127,
0.642442040715078));
#21774=CARTESIAN_POINT('Ctrl Pts',(0.109078032552995,-0.386717480603275,
0.640815160902589));
#21775=CARTESIAN_POINT('Ctrl Pts',(0.121846732641678,-0.417502809542364,
0.63851034608138));
#21776=CARTESIAN_POINT('Ctrl Pts',(0.125,-0.434262111007648,0.637867541108654));
#21777=CARTESIAN_POINT('Ctrl Pts',(0.125,-0.465737888992352,0.637867541108654));
#21778=CARTESIAN_POINT('Ctrl Pts',(0.121846732641678,-0.482497190457636,
0.63851034608138));
#21779=CARTESIAN_POINT('Ctrl Pts',(0.109078032552995,-0.513282519396725,
0.640815160902589));
#21780=CARTESIAN_POINT('Ctrl Pts',(0.099464669894764,-0.527312025401873,
0.642442040715078));
#21781=CARTESIAN_POINT('Ctrl Pts',(0.077312554408835,-0.549464140887802,
0.645482573914132));
#21782=CARTESIAN_POINT('Ctrl Pts',(0.0632828231545124,-0.559077918077178,
0.647096224417991));
#21783=CARTESIAN_POINT('Ctrl Pts',(0.0324967135411165,-0.571846918937749,
0.649370620646074));
#21784=CARTESIAN_POINT('Ctrl Pts',(0.0157371373481998,-0.575,0.65));
#21785=CARTESIAN_POINT('Ctrl Pts',(-1.38777878078145E-17,-0.575,0.65));
#21786=CARTESIAN_POINT('',(-0.125,-0.45,0.637867541108654));
#21787=CARTESIAN_POINT('Ctrl Pts',(-1.04083408558608E-17,-0.575,0.65));
#21788=CARTESIAN_POINT('Ctrl Pts',(-0.0157371373481998,-0.575,0.65));
#21789=CARTESIAN_POINT('Ctrl Pts',(-0.0324967135411164,-0.571846918937749,
0.649370620646074));
#21790=CARTESIAN_POINT('Ctrl Pts',(-0.0632828231545123,-0.559077918077178,
0.647096224417991));
#21791=CARTESIAN_POINT('Ctrl Pts',(-0.0773125544088349,-0.549464140887802,
0.645482573914132));
#21792=CARTESIAN_POINT('Ctrl Pts',(-0.099464669894764,-0.527312025401873,
0.642442040715078));
#21793=CARTESIAN_POINT('Ctrl Pts',(-0.109078032552995,-0.513282519396725,
0.640815160902589));
#21794=CARTESIAN_POINT('Ctrl Pts',(-0.121846732641678,-0.482497190457636,
0.63851034608138));
#21795=CARTESIAN_POINT('Ctrl Pts',(-0.125,-0.465737888992352,0.637867541108654));
#21796=CARTESIAN_POINT('Ctrl Pts',(-0.125,-0.45,0.637867541108654));
#21797=CARTESIAN_POINT('Ctrl Pts',(-0.125,-0.45,0.637867541108654));
#21798=CARTESIAN_POINT('Ctrl Pts',(-0.125,-0.434262111007648,0.637867541108654));
#21799=CARTESIAN_POINT('Ctrl Pts',(-0.121846732641678,-0.417502809542363,
0.63851034608138));
#21800=CARTESIAN_POINT('Ctrl Pts',(-0.109078032552995,-0.386717480603274,
0.640815160902589));
#21801=CARTESIAN_POINT('Ctrl Pts',(-0.0994646698947639,-0.372687974598127,
0.642442040715078));
#21802=CARTESIAN_POINT('Ctrl Pts',(-0.0773125544088348,-0.350535859112198,
0.645482573914132));
#21803=CARTESIAN_POINT('Ctrl Pts',(-0.0632828231545122,-0.340922081922822,
0.647096224417991));
#21804=CARTESIAN_POINT('Ctrl Pts',(-0.0324967135411163,-0.328153081062251,
0.649370620646074));
#21805=CARTESIAN_POINT('Ctrl Pts',(-0.0157371373481998,-0.325,0.65));
#21806=CARTESIAN_POINT('Ctrl Pts',(4.5102810375397E-17,-0.325,0.65));
#21807=CARTESIAN_POINT('Origin',(0.,-0.45,0.));
#21808=CARTESIAN_POINT('',(-0.125,-0.45,-0.379967103839267));
#21809=CARTESIAN_POINT('',(-0.125,-0.45,0.));
#21810=CARTESIAN_POINT('',(0.125,-0.45,-0.379967103839267));
#21811=CARTESIAN_POINT('Ctrl Pts',(0.125,-0.45,-0.379967103839267));
#21812=CARTESIAN_POINT('Ctrl Pts',(0.125,-0.465813100629203,-0.379967103839267));
#21813=CARTESIAN_POINT('Ctrl Pts',(0.121817958968287,-0.48260129709332,
-0.381057715344782));
#21814=CARTESIAN_POINT('Ctrl Pts',(0.109029967924066,-0.51336346023721,
-0.384911758361269));
#21815=CARTESIAN_POINT('Ctrl Pts',(0.0994291026068839,-0.527347592689753,
-0.38761064154154));
#21816=CARTESIAN_POINT('Ctrl Pts',(0.0773514949786257,-0.549425200318011,
-0.392612801026882));
#21817=CARTESIAN_POINT('Ctrl Pts',(0.0633657881355918,-0.559029081159106,
-0.395252954914593));
#21818=CARTESIAN_POINT('Ctrl Pts',(0.0325978607437828,-0.571819306519379,
-0.398970551469948));
#21819=CARTESIAN_POINT('Ctrl Pts',(0.0158075115832676,-0.575,-0.4));
#21820=CARTESIAN_POINT('Ctrl Pts',(-0.0158075115832676,-0.575,-0.4));
#21821=CARTESIAN_POINT('Ctrl Pts',(-0.0325978607437828,-0.571819306519379,
-0.398970551469948));
#21822=CARTESIAN_POINT('Ctrl Pts',(-0.0633657881355918,-0.559029081159106,
-0.395252954914593));
#21823=CARTESIAN_POINT('Ctrl Pts',(-0.0773514949786256,-0.549425200318011,
-0.392612801026882));
#21824=CARTESIAN_POINT('Ctrl Pts',(-0.0994291026068839,-0.527347592689753,
-0.38761064154154));
#21825=CARTESIAN_POINT('Ctrl Pts',(-0.109029967924066,-0.51336346023721,
-0.384911758361269));
#21826=CARTESIAN_POINT('Ctrl Pts',(-0.121817958968287,-0.48260129709332,
-0.381057715344782));
#21827=CARTESIAN_POINT('Ctrl Pts',(-0.125,-0.465813100629203,-0.379967103839267));
#21828=CARTESIAN_POINT('Ctrl Pts',(-0.125,-0.45,-0.379967103839267));
#21829=CARTESIAN_POINT('Ctrl Pts',(-0.125,-0.45,-0.379967103839267));
#21830=CARTESIAN_POINT('Ctrl Pts',(-0.125,-0.434186899370797,-0.379967103839267));
#21831=CARTESIAN_POINT('Ctrl Pts',(-0.121817958968287,-0.41739870290668,
-0.381057715344782));
#21832=CARTESIAN_POINT('Ctrl Pts',(-0.109029967924066,-0.38663653976279,
-0.384911758361269));
#21833=CARTESIAN_POINT('Ctrl Pts',(-0.0994291026068839,-0.372652407310247,
-0.38761064154154));
#21834=CARTESIAN_POINT('Ctrl Pts',(-0.0773514949786257,-0.350574799681989,
-0.392612801026882));
#21835=CARTESIAN_POINT('Ctrl Pts',(-0.0633657881355918,-0.340970918840894,
-0.395252954914593));
#21836=CARTESIAN_POINT('Ctrl Pts',(-0.0325978607437829,-0.328180693480621,
-0.398970551469948));
#21837=CARTESIAN_POINT('Ctrl Pts',(-0.0158075115832676,-0.325,-0.4));
#21838=CARTESIAN_POINT('Ctrl Pts',(0.0158075115832675,-0.325,-0.4));
#21839=CARTESIAN_POINT('Ctrl Pts',(0.0325978607437828,-0.328180693480621,
-0.398970551469948));
#21840=CARTESIAN_POINT('Ctrl Pts',(0.0633657881355917,-0.340970918840894,
-0.395252954914593));
#21841=CARTESIAN_POINT('Ctrl Pts',(0.0773514949786256,-0.350574799681989,
-0.392612801026882));
#21842=CARTESIAN_POINT('Ctrl Pts',(0.0994291026068839,-0.372652407310247,
-0.38761064154154));
#21843=CARTESIAN_POINT('Ctrl Pts',(0.109029967924066,-0.38663653976279,
-0.384911758361269));
#21844=CARTESIAN_POINT('Ctrl Pts',(0.121817958968287,-0.41739870290668,
-0.381057715344782));
#21845=CARTESIAN_POINT('Ctrl Pts',(0.125,-0.434186899370797,-0.379967103839267));
#21846=CARTESIAN_POINT('Ctrl Pts',(0.125,-0.45,-0.379967103839267));
#21847=CARTESIAN_POINT('Origin',(0.,-0.45,0.));
#21848=CARTESIAN_POINT('',(0.125,-0.45,0.379967103839267));
#21849=CARTESIAN_POINT('',(-0.125,-0.45,0.379967103839267));
#21850=CARTESIAN_POINT('Ctrl Pts',(0.125,-0.45,0.379967103839267));
#21851=CARTESIAN_POINT('Ctrl Pts',(0.125,-0.434186899370797,0.379967103839267));
#21852=CARTESIAN_POINT('Ctrl Pts',(0.121817958968287,-0.41739870290668,
0.381057715344782));
#21853=CARTESIAN_POINT('Ctrl Pts',(0.109029967924066,-0.38663653976279,
0.384911758361269));
#21854=CARTESIAN_POINT('Ctrl Pts',(0.0994291026068839,-0.372652407310247,
0.38761064154154));
#21855=CARTESIAN_POINT('Ctrl Pts',(0.0773514949786256,-0.350574799681989,
0.392612801026882));
#21856=CARTESIAN_POINT('Ctrl Pts',(0.0633657881355918,-0.340970918840894,
0.395252954914593));
#21857=CARTESIAN_POINT('Ctrl Pts',(0.0325978607437828,-0.328180693480621,
0.398970551469948));
#21858=CARTESIAN_POINT('Ctrl Pts',(0.0158075115832676,-0.325,0.4));
#21859=CARTESIAN_POINT('Ctrl Pts',(-0.0158075115832676,-0.325,0.4));
#21860=CARTESIAN_POINT('Ctrl Pts',(-0.0325978607437828,-0.328180693480621,
0.398970551469948));
#21861=CARTESIAN_POINT('Ctrl Pts',(-0.0633657881355918,-0.340970918840894,
0.395252954914593));
#21862=CARTESIAN_POINT('Ctrl Pts',(-0.0773514949786257,-0.350574799681989,
0.392612801026882));
#21863=CARTESIAN_POINT('Ctrl Pts',(-0.0994291026068839,-0.372652407310247,
0.38761064154154));
#21864=CARTESIAN_POINT('Ctrl Pts',(-0.109029967924066,-0.38663653976279,
0.384911758361269));
#21865=CARTESIAN_POINT('Ctrl Pts',(-0.121817958968287,-0.41739870290668,
0.381057715344782));
#21866=CARTESIAN_POINT('Ctrl Pts',(-0.125,-0.434186899370797,0.379967103839267));
#21867=CARTESIAN_POINT('Ctrl Pts',(-0.125,-0.45,0.379967103839267));
#21868=CARTESIAN_POINT('Ctrl Pts',(-0.125,-0.45,0.379967103839267));
#21869=CARTESIAN_POINT('Ctrl Pts',(-0.125,-0.465813100629203,0.379967103839267));
#21870=CARTESIAN_POINT('Ctrl Pts',(-0.121817958968287,-0.48260129709332,
0.381057715344782));
#21871=CARTESIAN_POINT('Ctrl Pts',(-0.109029967924066,-0.51336346023721,
0.384911758361269));
#21872=CARTESIAN_POINT('Ctrl Pts',(-0.0994291026068839,-0.527347592689753,
0.38761064154154));
#21873=CARTESIAN_POINT('Ctrl Pts',(-0.0773514949786256,-0.549425200318011,
0.392612801026882));
#21874=CARTESIAN_POINT('Ctrl Pts',(-0.0633657881355917,-0.559029081159106,
0.395252954914593));
#21875=CARTESIAN_POINT('Ctrl Pts',(-0.0325978607437828,-0.571819306519379,
0.398970551469948));
#21876=CARTESIAN_POINT('Ctrl Pts',(-0.0158075115832675,-0.575,0.4));
#21877=CARTESIAN_POINT('Ctrl Pts',(0.0158075115832676,-0.575,0.4));
#21878=CARTESIAN_POINT('Ctrl Pts',(0.0325978607437828,-0.571819306519379,
0.398970551469948));
#21879=CARTESIAN_POINT('Ctrl Pts',(0.0633657881355917,-0.559029081159106,
0.395252954914593));
#21880=CARTESIAN_POINT('Ctrl Pts',(0.0773514949786257,-0.549425200318011,
0.392612801026882));
#21881=CARTESIAN_POINT('Ctrl Pts',(0.0994291026068839,-0.527347592689753,
0.38761064154154));
#21882=CARTESIAN_POINT('Ctrl Pts',(0.109029967924066,-0.51336346023721,
0.384911758361269));
#21883=CARTESIAN_POINT('Ctrl Pts',(0.121817958968287,-0.48260129709332,
0.381057715344782));
#21884=CARTESIAN_POINT('Ctrl Pts',(0.125,-0.465813100629203,0.379967103839267));
#21885=CARTESIAN_POINT('Ctrl Pts',(0.125,-0.45,0.379967103839267));
#21886=CARTESIAN_POINT('',(-0.125,-0.45,0.));
#21887=CARTESIAN_POINT('Origin',(0.,0.,0.));
#21888=CARTESIAN_POINT('',(-0.4,-0.8,4.89858719658941E-17));
#21889=CARTESIAN_POINT('Origin',(0.,-0.8,0.));
#21890=CARTESIAN_POINT('',(-0.4,0.,4.89858719658941E-17));
#21891=CARTESIAN_POINT('',(-0.4,0.85,-4.89858719658941E-17));
#21892=CARTESIAN_POINT('',(-0.4,0.,4.89858719658941E-17));
#21893=CARTESIAN_POINT('Origin',(0.,0.85,0.));
#21894=CARTESIAN_POINT('Origin',(0.,-0.8,0.));
#21895=CARTESIAN_POINT('Origin',(0.,0.,0.));
#21896=CARTESIAN_POINT('',(-0.8,0.,9.79717439317883E-17));
#21897=CARTESIAN_POINT('Origin',(0.,0.,0.));
#21898=CARTESIAN_POINT('',(0.595438916863769,0.,0.137993139022126));
#21899=CARTESIAN_POINT('',(0.562830534889751,0.,0.238351419397483));
#21900=CARTESIAN_POINT('Origin',(0.562758945330873,0.,0.182851465569258));
#21901=CARTESIAN_POINT('',(0.523653836874034,0.,0.315240018494132));
#21902=CARTESIAN_POINT('Origin',(0.,0.,0.));
#21903=CARTESIAN_POINT('',(0.461629008549572,0.,0.40060987082025));
#21904=CARTESIAN_POINT('Origin',(0.478711351753049,0.,0.347804155687524));
#21905=CARTESIAN_POINT('',(0.40060987082025,0.,0.461629008549572));
#21906=CARTESIAN_POINT('Origin',(0.,0.,0.));
#21907=CARTESIAN_POINT('',(0.315240018494132,0.,0.523653836874034));
#21908=CARTESIAN_POINT('Origin',(0.347804155687523,0.,0.478711351753049));
#21909=CARTESIAN_POINT('',(0.238351419397483,0.,0.562830534889751));
#21910=CARTESIAN_POINT('Origin',(0.,0.,0.));
#21911=CARTESIAN_POINT('',(0.137993139022126,0.,0.595438916863769));
#21912=CARTESIAN_POINT('Origin',(0.182851465569258,0.,0.562758945330873));
#21913=CARTESIAN_POINT('',(0.0527614703521001,0.,0.608938287003997));
#21914=CARTESIAN_POINT('Origin',(0.,0.,0.));
#21915=CARTESIAN_POINT('',(-0.0527614703521003,0.,0.608938287003997));
#21916=CARTESIAN_POINT('Origin',(-1.08697158783324E-16,0.,0.591719772367581));
#21917=CARTESIAN_POINT('',(-0.137993139022126,0.,0.595438916863769));
#21918=CARTESIAN_POINT('Origin',(0.,0.,0.));
#21919=CARTESIAN_POINT('',(-0.238351419397483,0.,0.562830534889751));
#21920=CARTESIAN_POINT('Origin',(-0.182851465569258,0.,0.562758945330873));
#21921=CARTESIAN_POINT('',(-0.315240018494132,0.,0.523653836874034));
#21922=CARTESIAN_POINT('Origin',(0.,0.,0.));
#21923=CARTESIAN_POINT('',(-0.40060987082025,0.,0.461629008549572));
#21924=CARTESIAN_POINT('Origin',(-0.347804155687524,0.,0.478711351753049));
#21925=CARTESIAN_POINT('',(-0.461629008549572,0.,0.40060987082025));
#21926=CARTESIAN_POINT('Origin',(0.,0.,0.));
#21927=CARTESIAN_POINT('',(-0.523653836874034,0.,0.315240018494132));
#21928=CARTESIAN_POINT('Origin',(-0.478711351753049,0.,0.347804155687524));
#21929=CARTESIAN_POINT('',(-0.562830534889751,0.,0.238351419397483));
#21930=CARTESIAN_POINT('Origin',(0.,0.,0.));
#21931=CARTESIAN_POINT('',(-0.595438916863769,0.,0.137993139022126));
#21932=CARTESIAN_POINT('Origin',(-0.562758945330873,0.,0.182851465569258));
#21933=CARTESIAN_POINT('',(-0.608938287003997,0.,0.0527614703521002));
#21934=CARTESIAN_POINT('Origin',(0.,0.,0.));
#21935=CARTESIAN_POINT('',(-0.608938287003997,0.,-0.0527614703521003));
#21936=CARTESIAN_POINT('Origin',(-0.591719772367581,0.,-7.24647725222159E-17));
#21937=CARTESIAN_POINT('',(-0.595438916863769,0.,-0.137993139022126));
#21938=CARTESIAN_POINT('Origin',(0.,0.,0.));
#21939=CARTESIAN_POINT('',(-0.562830534889751,0.,-0.238351419397483));
#21940=CARTESIAN_POINT('Origin',(-0.562758945330873,0.,-0.182851465569258));
#21941=CARTESIAN_POINT('',(-0.523653836874034,0.,-0.315240018494132));
#21942=CARTESIAN_POINT('Origin',(0.,0.,0.));
#21943=CARTESIAN_POINT('',(-0.461629008549572,0.,-0.40060987082025));
#21944=CARTESIAN_POINT('Origin',(-0.478711351753049,0.,-0.347804155687524));
#21945=CARTESIAN_POINT('',(-0.40060987082025,0.,-0.461629008549572));
#21946=CARTESIAN_POINT('Origin',(0.,0.,0.));
#21947=CARTESIAN_POINT('',(-0.315240018494132,0.,-0.523653836874034));
#21948=CARTESIAN_POINT('Origin',(-0.347804155687524,0.,-0.478711351753049));
#21949=CARTESIAN_POINT('',(-0.238351419397483,0.,-0.562830534889751));
#21950=CARTESIAN_POINT('Origin',(0.,0.,0.));
#21951=CARTESIAN_POINT('',(-0.137993139022126,0.,-0.595438916863769));
#21952=CARTESIAN_POINT('Origin',(-0.182851465569258,0.,-0.562758945330873));
#21953=CARTESIAN_POINT('',(-0.0527614703521002,0.,-0.608938287003997));
#21954=CARTESIAN_POINT('Origin',(0.,0.,0.));
#21955=CARTESIAN_POINT('',(0.0527614703521003,0.,-0.608938287003997));
#21956=CARTESIAN_POINT('Origin',(3.6232386261108E-17,0.,-0.591719772367581));
#21957=CARTESIAN_POINT('',(0.137993139022126,0.,-0.595438916863769));
#21958=CARTESIAN_POINT('Origin',(0.,0.,0.));
#21959=CARTESIAN_POINT('',(0.238351419397483,0.,-0.562830534889751));
#21960=CARTESIAN_POINT('Origin',(0.182851465569258,0.,-0.562758945330873));
#21961=CARTESIAN_POINT('',(0.315240018494132,0.,-0.523653836874034));
#21962=CARTESIAN_POINT('Origin',(0.,0.,0.));
#21963=CARTESIAN_POINT('',(0.40060987082025,0.,-0.461629008549572));
#21964=CARTESIAN_POINT('Origin',(0.347804155687524,0.,-0.478711351753049));
#21965=CARTESIAN_POINT('',(0.461629008549572,0.,-0.40060987082025));
#21966=CARTESIAN_POINT('Origin',(0.,0.,0.));
#21967=CARTESIAN_POINT('',(0.523653836874034,0.,-0.315240018494132));
#21968=CARTESIAN_POINT('Origin',(0.478711351753049,0.,-0.347804155687524));
#21969=CARTESIAN_POINT('',(0.562830534889751,0.,-0.238351419397483));
#21970=CARTESIAN_POINT('Origin',(0.,0.,0.));
#21971=CARTESIAN_POINT('',(0.595438916863769,0.,-0.137993139022126));
#21972=CARTESIAN_POINT('Origin',(0.562758945330873,0.,-0.182851465569258));
#21973=CARTESIAN_POINT('',(0.608938287003997,0.,-0.0527614703521001));
#21974=CARTESIAN_POINT('Origin',(0.,0.,0.));
#21975=CARTESIAN_POINT('',(0.608938287003997,0.,0.0527614703521001));
#21976=CARTESIAN_POINT('Origin',(0.591719772367581,0.,0.));
#21977=CARTESIAN_POINT('Origin',(0.,0.,0.));
#21978=CARTESIAN_POINT('Origin',(0.,0.,0.));
#21979=CARTESIAN_POINT('',(-0.8,-0.1,9.79717439317883E-17));
#21980=CARTESIAN_POINT('Origin',(0.,-0.1,0.));
#21981=CARTESIAN_POINT('',(-0.8,0.,-9.79717439317883E-17));
#21982=CARTESIAN_POINT('Origin',(0.,-0.1,0.));
#21983=CARTESIAN_POINT('Origin',(0.,0.75,0.));
#21984=CARTESIAN_POINT('',(-0.8,0.75,9.79717439317883E-17));
#21985=CARTESIAN_POINT('Origin',(0.,0.75,0.));
#21986=CARTESIAN_POINT('',(0.562830534889751,0.75,0.238351419397483));
#21987=CARTESIAN_POINT('',(0.595438916863769,0.75,0.137993139022126));
#21988=CARTESIAN_POINT('Origin',(0.562758945330873,0.75,0.182851465569258));
#21989=CARTESIAN_POINT('',(0.608938287003997,0.75,0.0527614703521002));
#21990=CARTESIAN_POINT('Origin',(0.,0.75,0.));
#21991=CARTESIAN_POINT('',(0.608938287003997,0.75,-0.0527614703521002));
#21992=CARTESIAN_POINT('Origin',(0.591719772367581,0.75,0.));
#21993=CARTESIAN_POINT('',(0.595438916863769,0.75,-0.137993139022126));
#21994=CARTESIAN_POINT('Origin',(0.,0.75,0.));
#21995=CARTESIAN_POINT('',(0.562830534889751,0.75,-0.238351419397483));
#21996=CARTESIAN_POINT('Origin',(0.562758945330873,0.75,-0.182851465569258));
#21997=CARTESIAN_POINT('',(0.523653836874034,0.75,-0.315240018494132));
#21998=CARTESIAN_POINT('Origin',(0.,0.75,0.));
#21999=CARTESIAN_POINT('',(0.461629008549572,0.75,-0.40060987082025));
#22000=CARTESIAN_POINT('Origin',(0.478711351753049,0.75,-0.347804155687524));
#22001=CARTESIAN_POINT('',(0.40060987082025,0.75,-0.461629008549572));
#22002=CARTESIAN_POINT('Origin',(0.,0.75,0.));
#22003=CARTESIAN_POINT('',(0.315240018494132,0.75,-0.523653836874034));
#22004=CARTESIAN_POINT('Origin',(0.347804155687524,0.75,-0.478711351753049));
#22005=CARTESIAN_POINT('',(0.238351419397483,0.75,-0.562830534889751));
#22006=CARTESIAN_POINT('Origin',(0.,0.75,0.));
#22007=CARTESIAN_POINT('',(0.137993139022126,0.75,-0.595438916863769));
#22008=CARTESIAN_POINT('Origin',(0.182851465569258,0.75,-0.562758945330873));
#22009=CARTESIAN_POINT('',(0.0527614703521003,0.75,-0.608938287003997));
#22010=CARTESIAN_POINT('Origin',(0.,0.75,0.));
#22011=CARTESIAN_POINT('',(-0.0527614703521002,0.75,-0.608938287003997));
#22012=CARTESIAN_POINT('Origin',(3.6232386261108E-17,0.75,-0.591719772367581));
#22013=CARTESIAN_POINT('',(-0.137993139022126,0.75,-0.595438916863769));
#22014=CARTESIAN_POINT('Origin',(0.,0.75,0.));
#22015=CARTESIAN_POINT('',(-0.238351419397483,0.75,-0.562830534889751));
#22016=CARTESIAN_POINT('Origin',(-0.182851465569258,0.75,-0.562758945330873));
#22017=CARTESIAN_POINT('',(-0.315240018494132,0.75,-0.523653836874034));
#22018=CARTESIAN_POINT('Origin',(0.,0.75,0.));
#22019=CARTESIAN_POINT('',(-0.40060987082025,0.75,-0.461629008549572));
#22020=CARTESIAN_POINT('Origin',(-0.347804155687524,0.75,-0.478711351753049));
#22021=CARTESIAN_POINT('',(-0.461629008549572,0.75,-0.40060987082025));
#22022=CARTESIAN_POINT('Origin',(0.,0.75,0.));
#22023=CARTESIAN_POINT('',(-0.523653836874034,0.75,-0.315240018494132));
#22024=CARTESIAN_POINT('Origin',(-0.478711351753049,0.75,-0.347804155687524));
#22025=CARTESIAN_POINT('',(-0.562830534889751,0.75,-0.238351419397483));
#22026=CARTESIAN_POINT('Origin',(0.,0.75,0.));
#22027=CARTESIAN_POINT('',(-0.595438916863769,0.75,-0.137993139022126));
#22028=CARTESIAN_POINT('Origin',(-0.562758945330873,0.75,-0.182851465569258));
#22029=CARTESIAN_POINT('',(-0.608938287003997,0.75,-0.0527614703521003));
#22030=CARTESIAN_POINT('Origin',(0.,0.75,0.));
#22031=CARTESIAN_POINT('',(-0.608938287003997,0.75,0.0527614703521002));
#22032=CARTESIAN_POINT('Origin',(-0.591719772367581,0.75,-7.24647725222159E-17));
#22033=CARTESIAN_POINT('',(-0.595438916863769,0.75,0.137993139022126));
#22034=CARTESIAN_POINT('Origin',(0.,0.75,0.));
#22035=CARTESIAN_POINT('',(-0.562830534889751,0.75,0.238351419397483));
#22036=CARTESIAN_POINT('Origin',(-0.562758945330873,0.75,0.182851465569258));
#22037=CARTESIAN_POINT('',(-0.523653836874034,0.75,0.315240018494132));
#22038=CARTESIAN_POINT('Origin',(0.,0.75,0.));
#22039=CARTESIAN_POINT('',(-0.461629008549572,0.75,0.40060987082025));
#22040=CARTESIAN_POINT('Origin',(-0.478711351753049,0.75,0.347804155687524));
#22041=CARTESIAN_POINT('',(-0.40060987082025,0.75,0.461629008549572));
#22042=CARTESIAN_POINT('Origin',(0.,0.75,0.));
#22043=CARTESIAN_POINT('',(-0.315240018494132,0.75,0.523653836874034));
#22044=CARTESIAN_POINT('Origin',(-0.347804155687524,0.75,0.478711351753049));
#22045=CARTESIAN_POINT('',(-0.238351419397483,0.75,0.562830534889751));
#22046=CARTESIAN_POINT('Origin',(0.,0.75,0.));
#22047=CARTESIAN_POINT('',(-0.137993139022126,0.75,0.595438916863769));
#22048=CARTESIAN_POINT('Origin',(-0.182851465569258,0.75,0.562758945330873));
#22049=CARTESIAN_POINT('',(-0.0527614703521003,0.75,0.608938287003997));
#22050=CARTESIAN_POINT('Origin',(0.,0.75,0.));
#22051=CARTESIAN_POINT('',(0.0527614703521001,0.75,0.608938287003997));
#22052=CARTESIAN_POINT('Origin',(-1.08697158783324E-16,0.75,0.591719772367581));
#22053=CARTESIAN_POINT('',(0.137993139022126,0.75,0.595438916863769));
#22054=CARTESIAN_POINT('Origin',(0.,0.75,0.));
#22055=CARTESIAN_POINT('',(0.238351419397483,0.75,0.562830534889751));
#22056=CARTESIAN_POINT('Origin',(0.182851465569258,0.75,0.562758945330873));
#22057=CARTESIAN_POINT('',(0.315240018494132,0.75,0.523653836874034));
#22058=CARTESIAN_POINT('Origin',(0.,0.75,0.));
#22059=CARTESIAN_POINT('',(0.40060987082025,0.75,0.461629008549572));
#22060=CARTESIAN_POINT('Origin',(0.347804155687523,0.75,0.478711351753049));
#22061=CARTESIAN_POINT('',(0.461629008549572,0.75,0.40060987082025));
#22062=CARTESIAN_POINT('Origin',(0.,0.75,0.));
#22063=CARTESIAN_POINT('',(0.523653836874034,0.75,0.315240018494132));
#22064=CARTESIAN_POINT('Origin',(0.478711351753049,0.75,0.347804155687524));
#22065=CARTESIAN_POINT('Origin',(0.,0.75,0.));
#22066=CARTESIAN_POINT('Origin',(0.,0.75,0.));
#22067=CARTESIAN_POINT('',(-0.8,0.85,9.79717439317883E-17));
#22068=CARTESIAN_POINT('Origin',(0.,0.85,0.));
#22069=CARTESIAN_POINT('',(-0.8,0.75,9.79717439317883E-17));
#22070=CARTESIAN_POINT('Origin',(0.,0.85,0.));
#22071=CARTESIAN_POINT('Origin',(0.562758945330873,0.,0.182851465569258));
#22072=CARTESIAN_POINT('',(0.595438916863769,0.,0.137993139022126));
#22073=CARTESIAN_POINT('',(0.562830534889751,0.,0.238351419397483));
#22074=CARTESIAN_POINT('Origin',(0.,0.,0.));
#22075=CARTESIAN_POINT('',(0.523653836874034,0.,0.315240018494132));
#22076=CARTESIAN_POINT('Origin',(0.478711351753049,0.,0.347804155687524));
#22077=CARTESIAN_POINT('',(0.461629008549572,0.,0.40060987082025));
#22078=CARTESIAN_POINT('Origin',(0.,0.,0.));
#22079=CARTESIAN_POINT('',(0.40060987082025,0.,0.461629008549572));
#22080=CARTESIAN_POINT('Origin',(0.347804155687523,0.,0.478711351753049));
#22081=CARTESIAN_POINT('',(0.315240018494132,0.,0.523653836874034));
#22082=CARTESIAN_POINT('Origin',(0.,0.,0.));
#22083=CARTESIAN_POINT('',(0.238351419397483,0.,0.562830534889751));
#22084=CARTESIAN_POINT('Origin',(0.182851465569258,0.,0.562758945330873));
#22085=CARTESIAN_POINT('',(0.137993139022126,0.,0.595438916863769));
#22086=CARTESIAN_POINT('Origin',(0.,0.,0.));
#22087=CARTESIAN_POINT('',(0.0527614703521,0.,0.608938287003997));
#22088=CARTESIAN_POINT('Origin',(-1.08697158783324E-16,0.,0.591719772367581));
#22089=CARTESIAN_POINT('',(-0.0527614703521002,0.,0.608938287003997));
#22090=CARTESIAN_POINT('Origin',(0.,0.,0.));
#22091=CARTESIAN_POINT('',(-0.137993139022126,0.,0.595438916863769));
#22092=CARTESIAN_POINT('Origin',(-0.182851465569258,0.,0.562758945330873));
#22093=CARTESIAN_POINT('',(-0.238351419397483,0.,0.562830534889751));
#22094=CARTESIAN_POINT('Origin',(0.,0.,0.));
#22095=CARTESIAN_POINT('',(-0.315240018494132,0.,0.523653836874034));
#22096=CARTESIAN_POINT('Origin',(-0.347804155687524,0.,0.478711351753049));
#22097=CARTESIAN_POINT('',(-0.40060987082025,0.,0.461629008549572));
#22098=CARTESIAN_POINT('Origin',(0.,0.,0.));
#22099=CARTESIAN_POINT('',(-0.461629008549572,0.,0.40060987082025));
#22100=CARTESIAN_POINT('Origin',(-0.478711351753049,0.,0.347804155687524));
#22101=CARTESIAN_POINT('',(-0.523653836874034,0.,0.315240018494132));
#22102=CARTESIAN_POINT('Origin',(0.,0.,0.));
#22103=CARTESIAN_POINT('',(-0.562830534889751,0.,0.238351419397483));
#22104=CARTESIAN_POINT('Origin',(-0.562758945330873,0.,0.182851465569258));
#22105=CARTESIAN_POINT('',(-0.595438916863769,0.,0.137993139022126));
#22106=CARTESIAN_POINT('Origin',(0.,0.,0.));
#22107=CARTESIAN_POINT('',(-0.608938287003997,0.,0.0527614703521));
#22108=CARTESIAN_POINT('Origin',(-0.591719772367581,0.,-7.24647725222159E-17));
#22109=CARTESIAN_POINT('',(-0.608938287003997,0.,-0.0527614703521002));
#22110=CARTESIAN_POINT('Origin',(0.,0.,0.));
#22111=CARTESIAN_POINT('',(-0.595438916863769,0.,-0.137993139022126));
#22112=CARTESIAN_POINT('Origin',(-0.562758945330873,0.,-0.182851465569258));
#22113=CARTESIAN_POINT('',(-0.562830534889751,0.,-0.238351419397483));
#22114=CARTESIAN_POINT('Origin',(0.,0.,0.));
#22115=CARTESIAN_POINT('',(-0.523653836874034,0.,-0.315240018494132));
#22116=CARTESIAN_POINT('Origin',(-0.478711351753049,0.,-0.347804155687524));
#22117=CARTESIAN_POINT('',(-0.461629008549572,0.,-0.40060987082025));
#22118=CARTESIAN_POINT('Origin',(0.,0.,0.));
#22119=CARTESIAN_POINT('',(-0.40060987082025,0.,-0.461629008549572));
#22120=CARTESIAN_POINT('Origin',(-0.347804155687524,0.,-0.478711351753049));
#22121=CARTESIAN_POINT('',(-0.315240018494132,0.,-0.523653836874034));
#22122=CARTESIAN_POINT('Origin',(0.,0.,0.));
#22123=CARTESIAN_POINT('',(-0.238351419397483,0.,-0.562830534889751));
#22124=CARTESIAN_POINT('Origin',(-0.182851465569258,0.,-0.562758945330873));
#22125=CARTESIAN_POINT('',(-0.137993139022126,0.,-0.595438916863769));
#22126=CARTESIAN_POINT('Origin',(0.,0.,0.));
#22127=CARTESIAN_POINT('',(-0.0527614703521,0.,-0.608938287003997));
#22128=CARTESIAN_POINT('Origin',(3.6232386261108E-17,0.,-0.591719772367581));
#22129=CARTESIAN_POINT('',(0.0527614703521001,0.,-0.608938287003997));
#22130=CARTESIAN_POINT('Origin',(0.,0.,0.));
#22131=CARTESIAN_POINT('',(0.137993139022126,0.,-0.595438916863769));
#22132=CARTESIAN_POINT('Origin',(0.182851465569258,0.,-0.562758945330873));
#22133=CARTESIAN_POINT('',(0.238351419397483,0.,-0.562830534889751));
#22134=CARTESIAN_POINT('Origin',(0.,0.,0.));
#22135=CARTESIAN_POINT('',(0.315240018494132,0.,-0.523653836874034));
#22136=CARTESIAN_POINT('Origin',(0.347804155687524,0.,-0.478711351753049));
#22137=CARTESIAN_POINT('',(0.40060987082025,0.,-0.461629008549572));
#22138=CARTESIAN_POINT('Origin',(0.,0.,0.));
#22139=CARTESIAN_POINT('',(0.461629008549572,0.,-0.40060987082025));
#22140=CARTESIAN_POINT('Origin',(0.478711351753049,0.,-0.347804155687524));
#22141=CARTESIAN_POINT('',(0.523653836874034,0.,-0.315240018494132));
#22142=CARTESIAN_POINT('Origin',(0.,0.,0.));
#22143=CARTESIAN_POINT('',(0.562830534889751,0.,-0.238351419397483));
#22144=CARTESIAN_POINT('Origin',(0.562758945330873,0.,-0.182851465569258));
#22145=CARTESIAN_POINT('',(0.595438916863769,0.,-0.137993139022126));
#22146=CARTESIAN_POINT('Origin',(0.,0.,0.));
#22147=CARTESIAN_POINT('',(0.608938287003997,0.,0.0527614703521001));
#22148=CARTESIAN_POINT('Origin',(0.591719772367581,0.,0.));
#22149=CARTESIAN_POINT('',(0.608938287003997,0.,-0.0527614703521001));
#22150=CARTESIAN_POINT('Origin',(0.,0.,0.));
#23508=UNCERTAINTY_MEASURE_WITH_UNIT(LENGTH_MEASURE(0.001),#23588,
'DISTANCE_ACCURACY_VALUE',
'Maximum model space distance between geometric entities at asserted c
onnectivities');
#23522=UNCERTAINTY_MEASURE_WITH_UNIT(LENGTH_MEASURE(0.001),#23588,
'DISTANCE_ACCURACY_VALUE',
'Maximum model space distance between geometric entities at asserted c
onnectivities');
#23573=(
GEOMETRIC_REPRESENTATION_CONTEXT(3)
GLOBAL_UNCERTAINTY_ASSIGNED_CONTEXT((#23508))
GLOBAL_UNIT_ASSIGNED_CONTEXT((#23588,#23590,#23591))
REPRESENTATION_CONTEXT('','3D')
);
#23587=(
GEOMETRIC_REPRESENTATION_CONTEXT(3)
GLOBAL_UNCERTAINTY_ASSIGNED_CONTEXT((#23522))
GLOBAL_UNIT_ASSIGNED_CONTEXT((#23588,#23590,#23591))
REPRESENTATION_CONTEXT('','3D')
);
#23588=(
LENGTH_UNIT()
NAMED_UNIT(*)
SI_UNIT(.CENTI.,.METRE.)
);
#23590=(
NAMED_UNIT(*)
PLANE_ANGLE_UNIT()
SI_UNIT($,.RADIAN.)
);
#23591=(
NAMED_UNIT(*)
SI_UNIT($,.STERADIAN.)
SOLID_ANGLE_UNIT()
);
#23642=SHAPE_DEFINITION_REPRESENTATION(#23719,#23875);
#23719=PRODUCT_DEFINITION_SHAPE('',$,#23940);
#23875=SHAPE_REPRESENTATION('',(#13871),#23573);
#23889=PRODUCT_DEFINITION_CONTEXT('part definition',#24083,'design');
#23940=PRODUCT_DEFINITION(
'Timing Pulley - 2 mm Pitch, 20 Teeth, 8 mm Bore',
'Timing Pulley - 2 mm Pitch, 20 Teeth, 8 mm Bore',#24004,#23889);
#24004=PRODUCT_DEFINITION_FORMATION('',$,#24135);
#24083=APPLICATION_CONTEXT(
'Core Data for Automotive Mechanical Design Process');
#24084=PRODUCT_CONTEXT('part definition',#24083,'mechanical');
#24135=PRODUCT('Timing Pulley - 2 mm Pitch, 20 Teeth, 8 mm Bore',
'Timing Pulley - 2 mm Pitch, 20 Teeth, 8 mm Bore',
'Timing Pulley - 2 mm Pitch, 20 Teeth, 8 mm Bore',(#24084));
#24219=COLOUR_RGB('Off White',0.89,0.88,0.83);
#24220=FILL_AREA_STYLE_COLOUR('',#24219);
#24221=FILL_AREA_STYLE('',(#24220));
#24222=SURFACE_STYLE_FILL_AREA(#24221);
#24223=SURFACE_SIDE_STYLE('',(#24222));
#24224=SURFACE_STYLE_USAGE(.BOTH.,#24223);
#24225=PRESENTATION_STYLE_ASSIGNMENT((#24224));
ENDSEC;
END-ISO-10303-21;
